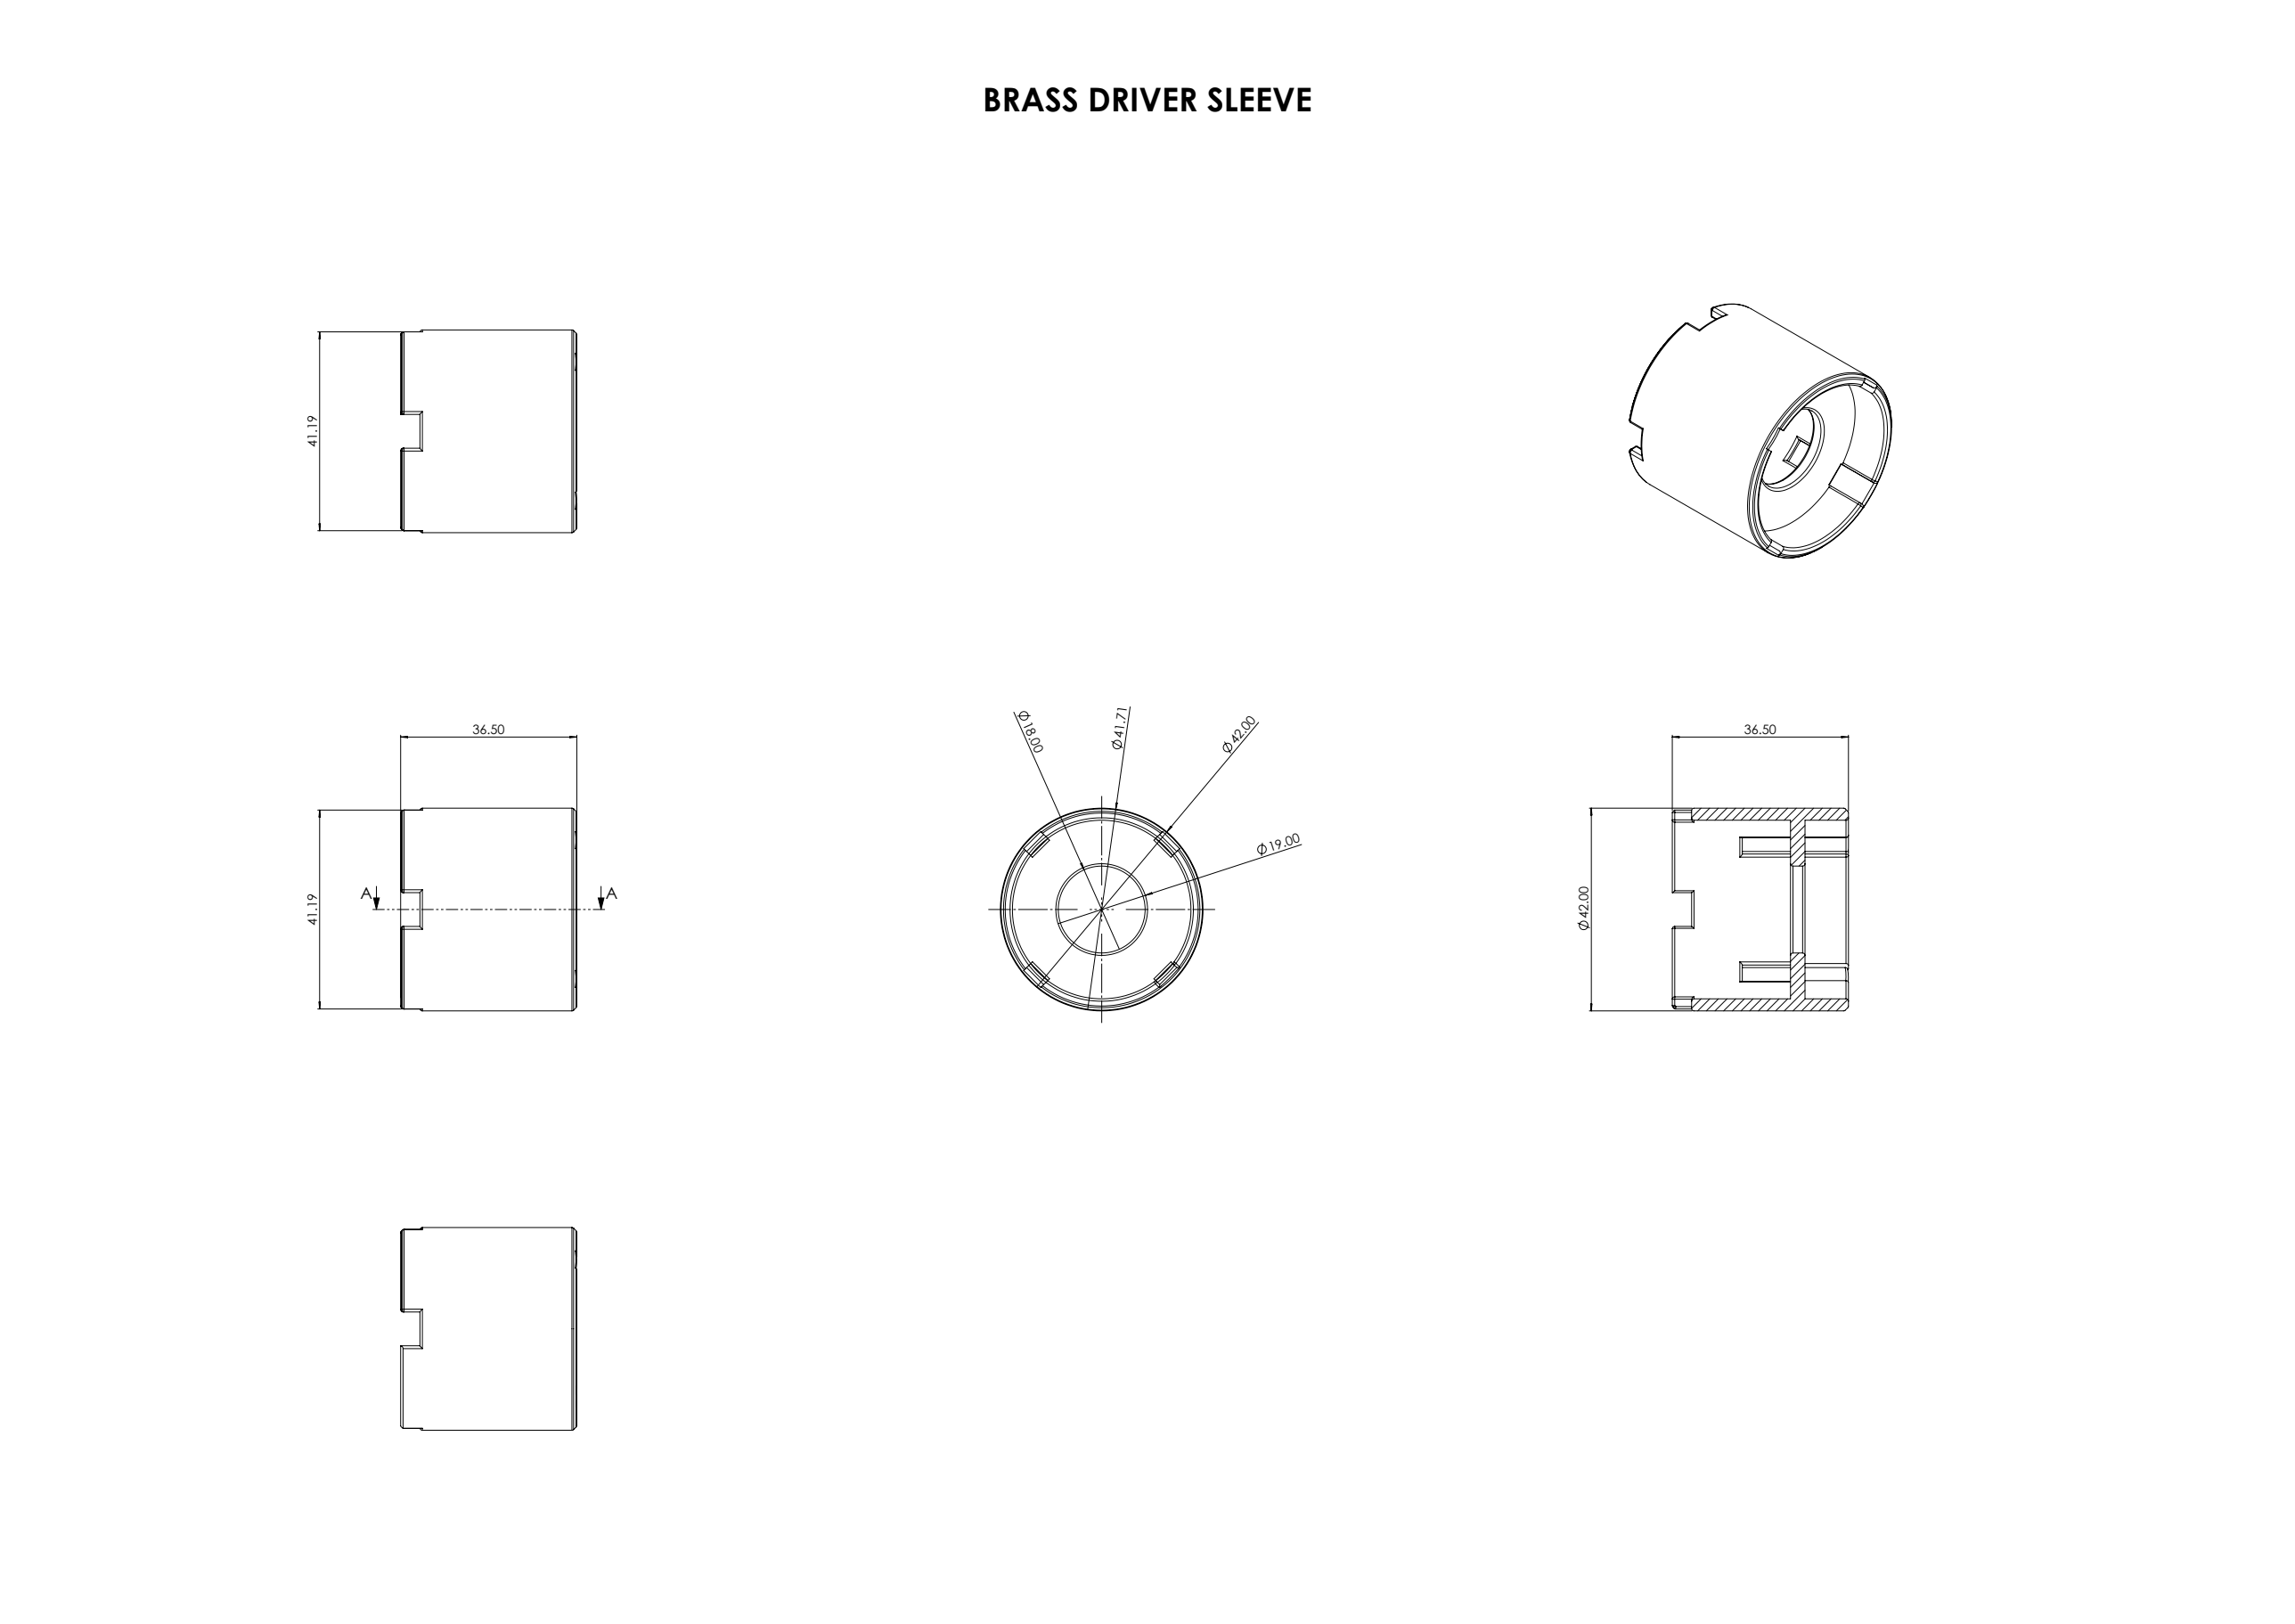
ISO-10303-21;
HEADER;
/* Generated by software containing ST-Developer
 * from STEP Tools, Inc. (www.steptools.com) 
 */

FILE_DESCRIPTION(
/* description */ (''),
/* implementation_level */ '2;1');

FILE_NAME(
/* name */ '11_Brass_Driver_Sleeve.step',
/* time_stamp */ '2026-10-11T13:00:10-07:00',
/* author */ (''),
/* organization */ (''),
/* preprocessor_version */ 'ST-DEVELOPER v20.2',
/* originating_system */ 'Autodesk Translation Framework v15.15.0.0',
/* authorisation */ '');

FILE_SCHEMA (('AUTOMOTIVE_DESIGN { 1 0 10303 214 3 1 1 }'));
ENDSEC;

DATA;
#10=MECHANICAL_DESIGN_GEOMETRIC_PRESENTATION_REPRESENTATION('',(#368),#65563);
#168=TOROIDAL_SURFACE('',#22042,9.5,0.5);
#169=TOROIDAL_SURFACE('',#22064,9.5,0.5);
#170=TOROIDAL_SURFACE('',#22095,20.2928932188135,0.5);
#171=TOROIDAL_SURFACE('',#22125,20.5,0.5);
#172=TOROIDAL_SURFACE('',#22149,20.5,0.5);
#173=TOROIDAL_SURFACE('',#22154,20.2928932188135,0.5);
#174=TOROIDAL_SURFACE('',#22157,20.5,0.5);
#175=TOROIDAL_SURFACE('',#22166,20.5,0.5);
#176=TOROIDAL_SURFACE('',#22186,20.5,0.5);
#177=TOROIDAL_SURFACE('',#22207,20.5,0.5);
#178=TOROIDAL_SURFACE('',#22220,20.5,0.5);
#179=TOROIDAL_SURFACE('',#22225,19.,0.5);
#180=TOROIDAL_SURFACE('',#22227,19.,0.5);
#181=TOROIDAL_SURFACE('',#22231,19.,0.5);
#182=TOROIDAL_SURFACE('',#22248,19.,0.5);
#183=TOROIDAL_SURFACE('',#22252,19.,0.5);
#184=TOROIDAL_SURFACE('',#22256,19.,0.5);
#185=TOROIDAL_SURFACE('',#22263,19.,0.5);
#186=TOROIDAL_SURFACE('',#22264,19.,0.5);
#187=TOROIDAL_SURFACE('',#22265,19.,0.5);
#188=TOROIDAL_SURFACE('',#22275,20.2928932188135,0.5);
#189=TOROIDAL_SURFACE('',#22289,19.,0.5);
#190=TOROIDAL_SURFACE('',#22299,19.,0.5);
#191=TOROIDAL_SURFACE('',#22302,20.5,0.5);
#192=TOROIDAL_SURFACE('',#22320,19.,0.5);
#193=TOROIDAL_SURFACE('',#22331,19.9928932188135,0.5);
#194=TOROIDAL_SURFACE('',#22335,19.,0.5);
#195=TOROIDAL_SURFACE('',#22338,19.9928932188135,0.5);
#196=TOROIDAL_SURFACE('',#22342,19.,0.5);
#197=TOROIDAL_SURFACE('',#22348,19.,0.5);
#198=TOROIDAL_SURFACE('',#22361,19.9928932188135,0.5);
#199=TOROIDAL_SURFACE('',#22372,19.,0.5);
#241=ELLIPSE('',#22319,0.707106781186544,0.5);
#242=ELLIPSE('',#22352,0.70710678118655,0.5);
#314=SPHERICAL_SURFACE('',#22100,0.5);
#315=SPHERICAL_SURFACE('',#22106,0.5);
#316=SPHERICAL_SURFACE('',#22109,0.5);
#317=SPHERICAL_SURFACE('',#22121,0.5);
#318=SPHERICAL_SURFACE('',#22142,0.5);
#319=SPHERICAL_SURFACE('',#22145,0.5);
#320=SPHERICAL_SURFACE('',#22162,0.5);
#321=SPHERICAL_SURFACE('',#22170,0.5);
#322=SPHERICAL_SURFACE('',#22173,0.5);
#323=SPHERICAL_SURFACE('',#22176,0.5);
#324=SPHERICAL_SURFACE('',#22191,0.5);
#325=SPHERICAL_SURFACE('',#22193,0.5);
#326=SPHERICAL_SURFACE('',#22200,0.5);
#327=SPHERICAL_SURFACE('',#22209,0.5);
#328=SPHERICAL_SURFACE('',#22217,0.5);
#329=SPHERICAL_SURFACE('',#22233,0.5);
#330=SPHERICAL_SURFACE('',#22259,0.5);
#331=SPHERICAL_SURFACE('',#22271,0.5);
#332=SPHERICAL_SURFACE('',#22282,0.500000000000002);
#333=SPHERICAL_SURFACE('',#22285,0.5);
#334=SPHERICAL_SURFACE('',#22324,0.5);
#335=SPHERICAL_SURFACE('',#22354,0.5);
#346=SHAPE_REPRESENTATION_RELATIONSHIP('SRR','None',#65624,#357);
#357=ADVANCED_BREP_SHAPE_REPRESENTATION('',(#379),#65562);
#368=STYLED_ITEM('',(#65802),#379);
#379=MANIFOLD_SOLID_BREP('Body1',#20018);
#495=CONICAL_SURFACE('',#22114,20.75,0.785398163397451);
#496=CONICAL_SURFACE('',#22152,20.75,0.785398163397451);
#497=CONICAL_SURFACE('',#22306,20.6,0.785398163397448);
#498=CONICAL_SURFACE('',#22380,20.75,0.785398163397451);
#499=CONICAL_SURFACE('',#22381,20.75,0.785398163397451);
#828=(
BOUNDED_CURVE()
B_SPLINE_CURVE(2,(#64727,#64728,#64729),.UNSPECIFIED.,.F.,.F.)
B_SPLINE_CURVE_WITH_KNOTS((3,3),(0.338124280435932,0.360943681531408),
 .UNSPECIFIED.)
CURVE()
GEOMETRIC_REPRESENTATION_ITEM()
RATIONAL_B_SPLINE_CURVE((1.00248873269084,1.00246071159709,1.00241757299052))
REPRESENTATION_ITEM('')
);
#829=(
BOUNDED_CURVE()
B_SPLINE_CURVE(2,(#64784,#64785,#64786),.UNSPECIFIED.,.F.,.F.)
B_SPLINE_CURVE_WITH_KNOTS((3,3),(0.230710993510061,0.25353039460556),
 .UNSPECIFIED.)
CURVE()
GEOMETRIC_REPRESENTATION_ITEM()
RATIONAL_B_SPLINE_CURVE((1.00241757299153,1.00246071159813,1.00248873269188))
REPRESENTATION_ITEM('')
);
#830=(
BOUNDED_CURVE()
B_SPLINE_CURVE(2,(#64793,#64794,#64795),.UNSPECIFIED.,.F.,.F.)
B_SPLINE_CURVE_WITH_KNOTS((3,3),(0.338124280435769,0.360943681531267),
 .UNSPECIFIED.)
CURVE()
GEOMETRIC_REPRESENTATION_ITEM()
RATIONAL_B_SPLINE_CURVE((1.00248873269167,1.00246071159791,1.00241757299132))
REPRESENTATION_ITEM('')
);
#831=(
BOUNDED_CURVE()
B_SPLINE_CURVE(2,(#64802,#64803,#64804),.UNSPECIFIED.,.F.,.F.)
B_SPLINE_CURVE_WITH_KNOTS((3,3),(0.230710993510149,0.253530394605615),
 .UNSPECIFIED.)
CURVE()
GEOMETRIC_REPRESENTATION_ITEM()
RATIONAL_B_SPLINE_CURVE((1.00241757299006,1.00246071159663,1.00248873269037))
REPRESENTATION_ITEM('')
);
#832=(
BOUNDED_CURVE()
B_SPLINE_CURVE(2,(#64812,#64813,#64814),.UNSPECIFIED.,.F.,.F.)
B_SPLINE_CURVE_WITH_KNOTS((3,3),(0.230710993510133,0.253530394605583),
 .UNSPECIFIED.)
CURVE()
GEOMETRIC_REPRESENTATION_ITEM()
RATIONAL_B_SPLINE_CURVE((1.00241757298939,1.00246071159594,1.00248873268967))
REPRESENTATION_ITEM('')
);
#833=(
BOUNDED_CURVE()
B_SPLINE_CURVE(2,(#64818,#64819,#64820),.UNSPECIFIED.,.F.,.F.)
B_SPLINE_CURVE_WITH_KNOTS((3,3),(0.338124280435993,0.360943681531517),
 .UNSPECIFIED.)
CURVE()
GEOMETRIC_REPRESENTATION_ITEM()
RATIONAL_B_SPLINE_CURVE((1.00248873269308,1.00246071159931,1.0024175729927))
REPRESENTATION_ITEM('')
);
#844=B_SPLINE_SURFACE_WITH_KNOTS('',3,3,((#63712,#63713,#63714,#63715),
(#63716,#63717,#63718,#63719),(#63720,#63721,#63722,#63723),(#63724,#63725,
#63726,#63727),(#63728,#63729,#63730,#63731),(#63732,#63733,#63734,#63735)),
 .UNSPECIFIED.,.F.,.F.,.F.,(4,1,1,4),(4,4),(0.,0.285714285714286,0.571428571428571,
1.),(0.143091562311917,0.172672323717935),.UNSPECIFIED.);
#845=B_SPLINE_SURFACE_WITH_KNOTS('',3,3,((#63754,#63755,#63756,#63757),
(#63758,#63759,#63760,#63761),(#63762,#63763,#63764,#63765),(#63766,#63767,
#63768,#63769),(#63770,#63771,#63772,#63773),(#63774,#63775,#63776,#63777)),
 .UNSPECIFIED.,.F.,.F.,.F.,(4,1,1,4),(4,4),(0.,0.285714285714286,0.571428571428571,
1.),(0.144052021996696,0.173632784471181),.UNSPECIFIED.);
#846=B_SPLINE_SURFACE_WITH_KNOTS('',3,3,((#63891,#63892,#63893,#63894),
(#63895,#63896,#63897,#63898),(#63899,#63900,#63901,#63902),(#63903,#63904,
#63905,#63906),(#63907,#63908,#63909,#63910),(#63911,#63912,#63913,#63914)),
 .UNSPECIFIED.,.F.,.F.,.F.,(4,1,1,4),(4,4),(0.,0.285714285714286,0.571428571428571,
1.),(0.357860307352845,0.38744106972591),.UNSPECIFIED.);
#847=B_SPLINE_SURFACE_WITH_KNOTS('',3,3,((#63991,#63992,#63993,#63994),
(#63995,#63996,#63997,#63998),(#63999,#64000,#64001,#64002),(#64003,#64004,
#64005,#64006),(#64007,#64008,#64009,#64010),(#64011,#64012,#64013,#64014)),
 .UNSPECIFIED.,.F.,.F.,.F.,(4,1,1,4),(4,4),(0.,0.285714285714286,0.571428571428571,
1.),(2.06363027950495E-16,0.0295807623344723),.UNSPECIFIED.);
#848=B_SPLINE_SURFACE_WITH_KNOTS('',3,3,((#64023,#64024,#64025,#64026),
(#64027,#64028,#64029,#64030),(#64031,#64032,#64033,#64034),(#64035,#64036,
#64037,#64038),(#64039,#64040,#64041,#64042),(#64043,#64044,#64045,#64046)),
 .UNSPECIFIED.,.F.,.F.,.F.,(4,1,1,4),(4,4),(0.,0.285714285714286,0.571428571428571,
1.),(6.08201692644882E-19,0.0295807623160019),.UNSPECIFIED.);
#849=B_SPLINE_SURFACE_WITH_KNOTS('',3,3,((#64167,#64168,#64169,#64170),
(#64171,#64172,#64173,#64174),(#64175,#64176,#64177,#64178),(#64179,#64180,
#64181,#64182),(#64183,#64184,#64185,#64186),(#64187,#64188,#64189,#64190)),
 .UNSPECIFIED.,.F.,.F.,.F.,(4,1,1,4),(4,4),(0.,0.285714285714286,0.571428571428571,
1.),(2.15031488595949E-16,0.0295807575131674),.UNSPECIFIED.);
#850=B_SPLINE_SURFACE_WITH_KNOTS('',3,3,((#65115,#65116,#65117,#65118),
(#65119,#65120,#65121,#65122),(#65123,#65124,#65125,#65126),(#65127,#65128,
#65129,#65130),(#65131,#65132,#65133,#65134),(#65135,#65136,#65137,#65138),
(#65139,#65140,#65141,#65142)),.UNSPECIFIED.,.F.,.F.,.F.,(4,1,1,1,4),(4,
4),(0.,0.285714285714286,0.571428571428571,0.857142857142857,1.),(0.82916884759973,
1.33025671401017),.UNSPECIFIED.);
#851=B_SPLINE_SURFACE_WITH_KNOTS('',3,3,((#65237,#65238,#65239,#65240),
(#65241,#65242,#65243,#65244),(#65245,#65246,#65247,#65248),(#65249,#65250,
#65251,#65252),(#65253,#65254,#65255,#65256),(#65257,#65258,#65259,#65260),
(#65261,#65262,#65263,#65264)),.UNSPECIFIED.,.F.,.F.,.F.,(4,1,1,1,4),(4,
4),(0.,0.285714285714286,0.571428571428571,0.857142857142857,1.),(0.829183372221167,
1.33027123863146),.UNSPECIFIED.);
#852=B_SPLINE_SURFACE_WITH_KNOTS('',3,3,((#65276,#65277,#65278,#65279),
(#65280,#65281,#65282,#65283),(#65284,#65285,#65286,#65287),(#65288,#65289,
#65290,#65291),(#65292,#65293,#65294,#65295),(#65296,#65297,#65298,#65299),
(#65300,#65301,#65302,#65303)),.UNSPECIFIED.,.F.,.F.,.F.,(4,1,1,1,4),(4,
4),(0.,0.285714285714286,0.571428571428571,0.857142857142857,1.),(0.829168847599735,
1.33025671401018),.UNSPECIFIED.);
#1040=PLANE('',#22050);
#1041=PLANE('',#22067);
#1042=PLANE('',#22077);
#1043=PLANE('',#22084);
#1044=PLANE('',#22091);
#1045=PLANE('',#22117);
#1046=PLANE('',#22123);
#1047=PLANE('',#22159);
#1048=PLANE('',#22183);
#1049=PLANE('',#22188);
#1050=PLANE('',#22197);
#1051=PLANE('',#22210);
#1052=PLANE('',#22213);
#1053=PLANE('',#22222);
#1054=PLANE('',#22250);
#1055=PLANE('',#22254);
#1056=PLANE('',#22267);
#1057=PLANE('',#22274);
#1058=PLANE('',#22278);
#1059=PLANE('',#22291);
#1060=PLANE('',#22292);
#1061=PLANE('',#22296);
#1062=PLANE('',#22298);
#1063=PLANE('',#22301);
#1064=PLANE('',#22312);
#1065=PLANE('',#22314);
#1066=PLANE('',#22316);
#1067=PLANE('',#22328);
#1068=PLANE('',#22330);
#1069=PLANE('',#22333);
#1070=PLANE('',#22337);
#1071=PLANE('',#22340);
#1072=PLANE('',#22344);
#1073=PLANE('',#22345);
#1074=PLANE('',#22358);
#1075=PLANE('',#22363);
#1076=PLANE('',#22366);
#1077=PLANE('',#22368);
#1078=PLANE('',#22374);
#1079=PLANE('',#22375);
#1080=PLANE('',#22376);
#1081=PLANE('',#22379);
#1124=FACE_BOUND('',#3382,.T.);
#1125=FACE_BOUND('',#3385,.T.);
#2151=FACE_OUTER_BOUND('',#3379,.T.);
#2152=FACE_OUTER_BOUND('',#3380,.T.);
#2153=FACE_OUTER_BOUND('',#3381,.T.);
#2154=FACE_OUTER_BOUND('',#3383,.T.);
#2155=FACE_OUTER_BOUND('',#3384,.T.);
#2156=FACE_OUTER_BOUND('',#3386,.T.);
#2157=FACE_OUTER_BOUND('',#3387,.T.);
#2158=FACE_OUTER_BOUND('',#3388,.T.);
#2159=FACE_OUTER_BOUND('',#3389,.T.);
#2160=FACE_OUTER_BOUND('',#3390,.T.);
#2161=FACE_OUTER_BOUND('',#3391,.T.);
#2162=FACE_OUTER_BOUND('',#3392,.T.);
#2163=FACE_OUTER_BOUND('',#3393,.T.);
#2164=FACE_OUTER_BOUND('',#3394,.T.);
#2165=FACE_OUTER_BOUND('',#3395,.T.);
#2166=FACE_OUTER_BOUND('',#3396,.T.);
#2167=FACE_OUTER_BOUND('',#3397,.T.);
#2168=FACE_OUTER_BOUND('',#3398,.T.);
#2169=FACE_OUTER_BOUND('',#3399,.T.);
#2170=FACE_OUTER_BOUND('',#3400,.T.);
#2171=FACE_OUTER_BOUND('',#3401,.T.);
#2172=FACE_OUTER_BOUND('',#3402,.T.);
#2173=FACE_OUTER_BOUND('',#3403,.T.);
#2174=FACE_OUTER_BOUND('',#3404,.T.);
#2175=FACE_OUTER_BOUND('',#3405,.T.);
#2176=FACE_OUTER_BOUND('',#3406,.T.);
#2177=FACE_OUTER_BOUND('',#3407,.T.);
#2178=FACE_OUTER_BOUND('',#3408,.T.);
#2179=FACE_OUTER_BOUND('',#3409,.T.);
#2180=FACE_OUTER_BOUND('',#3410,.T.);
#2181=FACE_OUTER_BOUND('',#3411,.T.);
#2182=FACE_OUTER_BOUND('',#3412,.T.);
#2183=FACE_OUTER_BOUND('',#3413,.T.);
#2184=FACE_OUTER_BOUND('',#3414,.T.);
#2185=FACE_OUTER_BOUND('',#3415,.T.);
#2186=FACE_OUTER_BOUND('',#3416,.T.);
#2187=FACE_OUTER_BOUND('',#3417,.T.);
#2188=FACE_OUTER_BOUND('',#3418,.T.);
#2189=FACE_OUTER_BOUND('',#3419,.T.);
#2190=FACE_OUTER_BOUND('',#3420,.T.);
#2191=FACE_OUTER_BOUND('',#3421,.T.);
#2192=FACE_OUTER_BOUND('',#3422,.T.);
#2193=FACE_OUTER_BOUND('',#3423,.T.);
#2194=FACE_OUTER_BOUND('',#3424,.T.);
#2195=FACE_OUTER_BOUND('',#3425,.T.);
#2196=FACE_OUTER_BOUND('',#3426,.T.);
#2197=FACE_OUTER_BOUND('',#3427,.T.);
#2198=FACE_OUTER_BOUND('',#3428,.T.);
#2199=FACE_OUTER_BOUND('',#3429,.T.);
#2200=FACE_OUTER_BOUND('',#3430,.T.);
#2201=FACE_OUTER_BOUND('',#3431,.T.);
#2202=FACE_OUTER_BOUND('',#3432,.T.);
#2203=FACE_OUTER_BOUND('',#3433,.T.);
#2204=FACE_OUTER_BOUND('',#3434,.T.);
#2205=FACE_OUTER_BOUND('',#3435,.T.);
#2206=FACE_OUTER_BOUND('',#3436,.T.);
#2207=FACE_OUTER_BOUND('',#3437,.T.);
#2208=FACE_OUTER_BOUND('',#3438,.T.);
#2209=FACE_OUTER_BOUND('',#3439,.T.);
#2210=FACE_OUTER_BOUND('',#3440,.T.);
#2211=FACE_OUTER_BOUND('',#3441,.T.);
#2212=FACE_OUTER_BOUND('',#3442,.T.);
#2213=FACE_OUTER_BOUND('',#3443,.T.);
#2214=FACE_OUTER_BOUND('',#3444,.T.);
#2215=FACE_OUTER_BOUND('',#3445,.T.);
#2216=FACE_OUTER_BOUND('',#3446,.T.);
#2217=FACE_OUTER_BOUND('',#3447,.T.);
#2218=FACE_OUTER_BOUND('',#3448,.T.);
#2219=FACE_OUTER_BOUND('',#3449,.T.);
#2220=FACE_OUTER_BOUND('',#3450,.T.);
#2221=FACE_OUTER_BOUND('',#3451,.T.);
#2222=FACE_OUTER_BOUND('',#3452,.T.);
#2223=FACE_OUTER_BOUND('',#3453,.T.);
#2224=FACE_OUTER_BOUND('',#3454,.T.);
#2225=FACE_OUTER_BOUND('',#3455,.T.);
#2226=FACE_OUTER_BOUND('',#3456,.T.);
#2227=FACE_OUTER_BOUND('',#3457,.T.);
#2228=FACE_OUTER_BOUND('',#3458,.T.);
#2229=FACE_OUTER_BOUND('',#3459,.T.);
#2230=FACE_OUTER_BOUND('',#3460,.T.);
#2231=FACE_OUTER_BOUND('',#3461,.T.);
#2232=FACE_OUTER_BOUND('',#3462,.T.);
#2233=FACE_OUTER_BOUND('',#3463,.T.);
#2234=FACE_OUTER_BOUND('',#3464,.T.);
#2235=FACE_OUTER_BOUND('',#3465,.T.);
#2236=FACE_OUTER_BOUND('',#3466,.T.);
#2237=FACE_OUTER_BOUND('',#3467,.T.);
#2238=FACE_OUTER_BOUND('',#3468,.T.);
#2239=FACE_OUTER_BOUND('',#3469,.T.);
#2240=FACE_OUTER_BOUND('',#3470,.T.);
#2241=FACE_OUTER_BOUND('',#3471,.T.);
#2242=FACE_OUTER_BOUND('',#3472,.T.);
#2243=FACE_OUTER_BOUND('',#3473,.T.);
#2244=FACE_OUTER_BOUND('',#3474,.T.);
#2245=FACE_OUTER_BOUND('',#3475,.T.);
#2246=FACE_OUTER_BOUND('',#3476,.T.);
#2247=FACE_OUTER_BOUND('',#3477,.T.);
#2248=FACE_OUTER_BOUND('',#3478,.T.);
#2249=FACE_OUTER_BOUND('',#3479,.T.);
#2250=FACE_OUTER_BOUND('',#3480,.T.);
#2251=FACE_OUTER_BOUND('',#3481,.T.);
#2252=FACE_OUTER_BOUND('',#3482,.T.);
#2253=FACE_OUTER_BOUND('',#3483,.T.);
#2254=FACE_OUTER_BOUND('',#3484,.T.);
#2255=FACE_OUTER_BOUND('',#3485,.T.);
#2256=FACE_OUTER_BOUND('',#3486,.T.);
#2257=FACE_OUTER_BOUND('',#3487,.T.);
#2258=FACE_OUTER_BOUND('',#3488,.T.);
#2259=FACE_OUTER_BOUND('',#3489,.T.);
#2260=FACE_OUTER_BOUND('',#3490,.T.);
#2261=FACE_OUTER_BOUND('',#3491,.T.);
#2262=FACE_OUTER_BOUND('',#3492,.T.);
#2263=FACE_OUTER_BOUND('',#3493,.T.);
#2264=FACE_OUTER_BOUND('',#3494,.T.);
#2265=FACE_OUTER_BOUND('',#3495,.T.);
#2266=FACE_OUTER_BOUND('',#3496,.T.);
#2267=FACE_OUTER_BOUND('',#3497,.T.);
#2268=FACE_OUTER_BOUND('',#3498,.T.);
#2269=FACE_OUTER_BOUND('',#3499,.T.);
#2270=FACE_OUTER_BOUND('',#3500,.T.);
#2271=FACE_OUTER_BOUND('',#3501,.T.);
#2272=FACE_OUTER_BOUND('',#3502,.T.);
#2273=FACE_OUTER_BOUND('',#3503,.T.);
#2274=FACE_OUTER_BOUND('',#3504,.T.);
#2275=FACE_OUTER_BOUND('',#3505,.T.);
#2276=FACE_OUTER_BOUND('',#3506,.T.);
#2277=FACE_OUTER_BOUND('',#3507,.T.);
#2278=FACE_OUTER_BOUND('',#3508,.T.);
#2279=FACE_OUTER_BOUND('',#3509,.T.);
#2280=FACE_OUTER_BOUND('',#3510,.T.);
#2281=FACE_OUTER_BOUND('',#3511,.T.);
#2282=FACE_OUTER_BOUND('',#3512,.T.);
#2283=FACE_OUTER_BOUND('',#3513,.T.);
#2284=FACE_OUTER_BOUND('',#3514,.T.);
#2285=FACE_OUTER_BOUND('',#3515,.T.);
#2286=FACE_OUTER_BOUND('',#3516,.T.);
#2287=FACE_OUTER_BOUND('',#3517,.T.);
#2288=FACE_OUTER_BOUND('',#3518,.T.);
#2289=FACE_OUTER_BOUND('',#3519,.T.);
#2290=FACE_OUTER_BOUND('',#3520,.T.);
#2291=FACE_OUTER_BOUND('',#3521,.T.);
#2292=FACE_OUTER_BOUND('',#3522,.T.);
#2293=FACE_OUTER_BOUND('',#3523,.T.);
#2294=FACE_OUTER_BOUND('',#3524,.T.);
#2295=FACE_OUTER_BOUND('',#3525,.T.);
#2296=FACE_OUTER_BOUND('',#3526,.T.);
#2297=FACE_OUTER_BOUND('',#3527,.T.);
#2298=FACE_OUTER_BOUND('',#3528,.T.);
#2299=FACE_OUTER_BOUND('',#3529,.T.);
#2300=FACE_OUTER_BOUND('',#3530,.T.);
#2301=FACE_OUTER_BOUND('',#3531,.T.);
#2302=FACE_OUTER_BOUND('',#3532,.T.);
#2303=FACE_OUTER_BOUND('',#3533,.T.);
#2304=FACE_OUTER_BOUND('',#3534,.T.);
#2305=FACE_OUTER_BOUND('',#3535,.T.);
#2306=FACE_OUTER_BOUND('',#3536,.T.);
#2307=FACE_OUTER_BOUND('',#3537,.T.);
#2308=FACE_OUTER_BOUND('',#3538,.T.);
#2309=FACE_OUTER_BOUND('',#3539,.T.);
#2310=FACE_OUTER_BOUND('',#3540,.T.);
#2311=FACE_OUTER_BOUND('',#3541,.T.);
#3379=EDGE_LOOP('',(#17440,#17441,#17442,#17443,#17444));
#3380=EDGE_LOOP('',(#17445,#17446,#17447,#17448,#17449,#17450));
#3381=EDGE_LOOP('',(#17451,#17452,#17453,#17454,#17455,#17456,#17457,#17458,
#17459,#17460,#17461,#17462,#17463,#17464,#17465,#17466,#17467,#17468,#17469,
#17470,#17471,#17472,#17473,#17474,#17475));
#3382=EDGE_LOOP('',(#17476));
#3383=EDGE_LOOP('',(#17477,#17478,#17479,#17480,#17481));
#3384=EDGE_LOOP('',(#17482,#17483,#17484,#17485,#17486,#17487,#17488,#17489,
#17490,#17491,#17492,#17493,#17494,#17495,#17496,#17497,#17498,#17499));
#3385=EDGE_LOOP('',(#17500));
#3386=EDGE_LOOP('',(#17501,#17502,#17503,#17504));
#3387=EDGE_LOOP('',(#17505,#17506,#17507,#17508));
#3388=EDGE_LOOP('',(#17509,#17510,#17511,#17512));
#3389=EDGE_LOOP('',(#17513,#17514,#17515,#17516));
#3390=EDGE_LOOP('',(#17517,#17518,#17519,#17520));
#3391=EDGE_LOOP('',(#17521,#17522,#17523,#17524));
#3392=EDGE_LOOP('',(#17525,#17526,#17527,#17528));
#3393=EDGE_LOOP('',(#17529,#17530,#17531,#17532));
#3394=EDGE_LOOP('',(#17533,#17534,#17535,#17536));
#3395=EDGE_LOOP('',(#17537,#17538,#17539,#17540));
#3396=EDGE_LOOP('',(#17541,#17542,#17543));
#3397=EDGE_LOOP('',(#17544,#17545,#17546,#17547));
#3398=EDGE_LOOP('',(#17548,#17549,#17550));
#3399=EDGE_LOOP('',(#17551,#17552,#17553));
#3400=EDGE_LOOP('',(#17554,#17555,#17556,#17557));
#3401=EDGE_LOOP('',(#17558,#17559,#17560,#17561));
#3402=EDGE_LOOP('',(#17562,#17563,#17564,#17565));
#3403=EDGE_LOOP('',(#17566,#17567,#17568,#17569));
#3404=EDGE_LOOP('',(#17570,#17571,#17572,#17573,#17574,#17575));
#3405=EDGE_LOOP('',(#17576,#17577,#17578,#17579,#17580));
#3406=EDGE_LOOP('',(#17581,#17582,#17583));
#3407=EDGE_LOOP('',(#17584,#17585,#17586,#17587));
#3408=EDGE_LOOP('',(#17588,#17589,#17590,#17591));
#3409=EDGE_LOOP('',(#17592,#17593,#17594,#17595,#17596,#17597,#17598,#17599,
#17600,#17601,#17602,#17603,#17604,#17605,#17606,#17607,#17608,#17609,#17610,
#17611,#17612));
#3410=EDGE_LOOP('',(#17613,#17614,#17615,#17616,#17617));
#3411=EDGE_LOOP('',(#17618,#17619,#17620));
#3412=EDGE_LOOP('',(#17621,#17622,#17623));
#3413=EDGE_LOOP('',(#17624,#17625,#17626,#17627));
#3414=EDGE_LOOP('',(#17628,#17629,#17630,#17631));
#3415=EDGE_LOOP('',(#17632,#17633,#17634,#17635));
#3416=EDGE_LOOP('',(#17636,#17637,#17638,#17639));
#3417=EDGE_LOOP('',(#17640,#17641,#17642,#17643));
#3418=EDGE_LOOP('',(#17644,#17645,#17646,#17647,#17648,#17649));
#3419=EDGE_LOOP('',(#17650,#17651,#17652));
#3420=EDGE_LOOP('',(#17653,#17654,#17655,#17656));
#3421=EDGE_LOOP('',(#17657,#17658,#17659));
#3422=EDGE_LOOP('',(#17660,#17661,#17662));
#3423=EDGE_LOOP('',(#17663,#17664,#17665));
#3424=EDGE_LOOP('',(#17666,#17667,#17668,#17669));
#3425=EDGE_LOOP('',(#17670,#17671,#17672,#17673));
#3426=EDGE_LOOP('',(#17674,#17675,#17676,#17677,#17678));
#3427=EDGE_LOOP('',(#17679,#17680,#17681,#17682,#17683));
#3428=EDGE_LOOP('',(#17684,#17685,#17686,#17687,#17688,#17689));
#3429=EDGE_LOOP('',(#17690,#17691,#17692,#17693));
#3430=EDGE_LOOP('',(#17694,#17695,#17696,#17697,#17698));
#3431=EDGE_LOOP('',(#17699,#17700,#17701,#17702,#17703,#17704));
#3432=EDGE_LOOP('',(#17705,#17706,#17707));
#3433=EDGE_LOOP('',(#17708,#17709,#17710));
#3434=EDGE_LOOP('',(#17711,#17712,#17713,#17714));
#3435=EDGE_LOOP('',(#17715,#17716,#17717,#17718,#17719,#17720));
#3436=EDGE_LOOP('',(#17721,#17722,#17723,#17724,#17725));
#3437=EDGE_LOOP('',(#17726,#17727,#17728));
#3438=EDGE_LOOP('',(#17729,#17730,#17731,#17732));
#3439=EDGE_LOOP('',(#17733,#17734,#17735,#17736,#17737));
#3440=EDGE_LOOP('',(#17738,#17739,#17740,#17741));
#3441=EDGE_LOOP('',(#17742,#17743,#17744));
#3442=EDGE_LOOP('',(#17745,#17746,#17747,#17748,#17749,#17750));
#3443=EDGE_LOOP('',(#17751,#17752,#17753,#17754));
#3444=EDGE_LOOP('',(#17755,#17756,#17757,#17758));
#3445=EDGE_LOOP('',(#17759,#17760,#17761,#17762));
#3446=EDGE_LOOP('',(#17763,#17764,#17765));
#3447=EDGE_LOOP('',(#17766,#17767,#17768,#17769));
#3448=EDGE_LOOP('',(#17770,#17771,#17772,#17773,#17774,#17775));
#3449=EDGE_LOOP('',(#17776,#17777,#17778,#17779,#17780,#17781));
#3450=EDGE_LOOP('',(#17782,#17783,#17784,#17785));
#3451=EDGE_LOOP('',(#17786,#17787,#17788,#17789));
#3452=EDGE_LOOP('',(#17790,#17791,#17792,#17793,#17794,#17795));
#3453=EDGE_LOOP('',(#17796,#17797,#17798));
#3454=EDGE_LOOP('',(#17799,#17800,#17801,#17802));
#3455=EDGE_LOOP('',(#17803,#17804,#17805,#17806,#17807,#17808,#17809,#17810,
#17811,#17812,#17813,#17814,#17815,#17816,#17817,#17818,#17819,#17820,#17821,
#17822,#17823,#17824,#17825,#17826,#17827,#17828,#17829,#17830,#17831,#17832,
#17833,#17834,#17835,#17836,#17837,#17838));
#3456=EDGE_LOOP('',(#17839,#17840,#17841,#17842));
#3457=EDGE_LOOP('',(#17843,#17844,#17845,#17846,#17847,#17848));
#3458=EDGE_LOOP('',(#17849,#17850,#17851,#17852));
#3459=EDGE_LOOP('',(#17853,#17854,#17855,#17856));
#3460=EDGE_LOOP('',(#17857,#17858,#17859,#17860,#17861,#17862));
#3461=EDGE_LOOP('',(#17863,#17864,#17865,#17866));
#3462=EDGE_LOOP('',(#17867,#17868,#17869,#17870));
#3463=EDGE_LOOP('',(#17871,#17872,#17873,#17874,#17875));
#3464=EDGE_LOOP('',(#17876,#17877,#17878));
#3465=EDGE_LOOP('',(#17879,#17880,#17881,#17882));
#3466=EDGE_LOOP('',(#17883,#17884,#17885,#17886,#17887,#17888,#17889));
#3467=EDGE_LOOP('',(#17890,#17891,#17892,#17893));
#3468=EDGE_LOOP('',(#17894,#17895,#17896,#17897,#17898,#17899));
#3469=EDGE_LOOP('',(#17900,#17901,#17902,#17903,#17904,#17905));
#3470=EDGE_LOOP('',(#17906,#17907,#17908,#17909));
#3471=EDGE_LOOP('',(#17910,#17911,#17912,#17913));
#3472=EDGE_LOOP('',(#17914,#17915,#17916));
#3473=EDGE_LOOP('',(#17917,#17918,#17919,#17920,#17921));
#3474=EDGE_LOOP('',(#17922,#17923,#17924,#17925,#17926));
#3475=EDGE_LOOP('',(#17927,#17928,#17929,#17930));
#3476=EDGE_LOOP('',(#17931,#17932,#17933,#17934));
#3477=EDGE_LOOP('',(#17935,#17936,#17937,#17938));
#3478=EDGE_LOOP('',(#17939,#17940,#17941));
#3479=EDGE_LOOP('',(#17942,#17943,#17944));
#3480=EDGE_LOOP('',(#17945,#17946,#17947,#17948));
#3481=EDGE_LOOP('',(#17949,#17950,#17951,#17952));
#3482=EDGE_LOOP('',(#17953,#17954,#17955,#17956));
#3483=EDGE_LOOP('',(#17957,#17958,#17959,#17960,#17961,#17962));
#3484=EDGE_LOOP('',(#17963,#17964,#17965,#17966,#17967));
#3485=EDGE_LOOP('',(#17968,#17969,#17970,#17971,#17972,#17973));
#3486=EDGE_LOOP('',(#17974,#17975,#17976,#17977,#17978,#17979));
#3487=EDGE_LOOP('',(#17980,#17981,#17982,#17983));
#3488=EDGE_LOOP('',(#17984,#17985,#17986,#17987,#17988,#17989,#17990,#17991,
#17992,#17993,#17994,#17995,#17996,#17997,#17998));
#3489=EDGE_LOOP('',(#17999,#18000,#18001,#18002,#18003,#18004));
#3490=EDGE_LOOP('',(#18005,#18006,#18007,#18008));
#3491=EDGE_LOOP('',(#18009,#18010,#18011,#18012,#18013,#18014));
#3492=EDGE_LOOP('',(#18015,#18016,#18017,#18018,#18019,#18020,#18021,#18022,
#18023,#18024,#18025,#18026,#18027,#18028,#18029,#18030,#18031));
#3493=EDGE_LOOP('',(#18032,#18033,#18034,#18035));
#3494=EDGE_LOOP('',(#18036,#18037,#18038,#18039,#18040,#18041,#18042,#18043,
#18044,#18045,#18046,#18047,#18048,#18049,#18050));
#3495=EDGE_LOOP('',(#18051,#18052,#18053,#18054));
#3496=EDGE_LOOP('',(#18055,#18056,#18057,#18058,#18059,#18060,#18061,#18062,
#18063,#18064,#18065,#18066,#18067,#18068,#18069));
#3497=EDGE_LOOP('',(#18070,#18071,#18072,#18073));
#3498=EDGE_LOOP('',(#18074,#18075,#18076,#18077,#18078,#18079,#18080,#18081,
#18082,#18083,#18084,#18085,#18086,#18087,#18088));
#3499=EDGE_LOOP('',(#18089,#18090,#18091,#18092,#18093));
#3500=EDGE_LOOP('',(#18094,#18095,#18096,#18097));
#3501=EDGE_LOOP('',(#18098,#18099,#18100));
#3502=EDGE_LOOP('',(#18101,#18102,#18103,#18104));
#3503=EDGE_LOOP('',(#18105,#18106,#18107,#18108));
#3504=EDGE_LOOP('',(#18109,#18110,#18111,#18112));
#3505=EDGE_LOOP('',(#18113,#18114,#18115,#18116));
#3506=EDGE_LOOP('',(#18117,#18118,#18119,#18120));
#3507=EDGE_LOOP('',(#18121,#18122,#18123,#18124));
#3508=EDGE_LOOP('',(#18125,#18126,#18127,#18128));
#3509=EDGE_LOOP('',(#18129,#18130,#18131,#18132));
#3510=EDGE_LOOP('',(#18133,#18134,#18135,#18136));
#3511=EDGE_LOOP('',(#18137,#18138,#18139,#18140));
#3512=EDGE_LOOP('',(#18141,#18142,#18143,#18144));
#3513=EDGE_LOOP('',(#18145,#18146,#18147,#18148));
#3514=EDGE_LOOP('',(#18149,#18150,#18151,#18152));
#3515=EDGE_LOOP('',(#18153,#18154,#18155,#18156));
#3516=EDGE_LOOP('',(#18157,#18158,#18159,#18160));
#3517=EDGE_LOOP('',(#18161,#18162,#18163,#18164));
#3518=EDGE_LOOP('',(#18165,#18166,#18167,#18168));
#3519=EDGE_LOOP('',(#18169,#18170,#18171,#18172,#18173));
#3520=EDGE_LOOP('',(#18174,#18175,#18176));
#3521=EDGE_LOOP('',(#18177,#18178,#18179,#18180));
#3522=EDGE_LOOP('',(#18181,#18182,#18183,#18184));
#3523=EDGE_LOOP('',(#18185,#18186,#18187,#18188,#18189,#18190,#18191,#18192,
#18193,#18194,#18195));
#3524=EDGE_LOOP('',(#18196,#18197,#18198,#18199,#18200,#18201,#18202,#18203,
#18204,#18205,#18206));
#3525=EDGE_LOOP('',(#18207,#18208,#18209,#18210,#18211,#18212));
#3526=EDGE_LOOP('',(#18213,#18214,#18215,#18216,#18217,#18218,#18219,#18220,
#18221,#18222,#18223));
#3527=EDGE_LOOP('',(#18224,#18225,#18226,#18227));
#3528=EDGE_LOOP('',(#18228,#18229,#18230,#18231));
#3529=EDGE_LOOP('',(#18232,#18233,#18234,#18235));
#3530=EDGE_LOOP('',(#18236,#18237,#18238,#18239));
#3531=EDGE_LOOP('',(#18240,#18241,#18242,#18243));
#3532=EDGE_LOOP('',(#18244,#18245,#18246,#18247));
#3533=EDGE_LOOP('',(#18248,#18249,#18250,#18251,#18252,#18253));
#3534=EDGE_LOOP('',(#18254,#18255,#18256,#18257));
#3535=EDGE_LOOP('',(#18258,#18259,#18260,#18261,#18262,#18263,#18264,#18265,
#18266,#18267,#18268,#18269,#18270,#18271,#18272));
#3536=EDGE_LOOP('',(#18273,#18274,#18275,#18276,#18277,#18278,#18279,#18280,
#18281,#18282,#18283,#18284,#18285,#18286,#18287));
#3537=EDGE_LOOP('',(#18288,#18289,#18290,#18291));
#3538=EDGE_LOOP('',(#18292,#18293,#18294,#18295));
#3539=EDGE_LOOP('',(#18296,#18297,#18298,#18299,#18300,#18301));
#3540=EDGE_LOOP('',(#18302,#18303,#18304,#18305));
#3541=EDGE_LOOP('',(#18306,#18307,#18308,#18309));
#4483=CIRCLE('',#22043,9.5);
#4484=CIRCLE('',#22044,0.5);
#4485=CIRCLE('',#22045,9.);
#4486=CIRCLE('',#22046,9.);
#4487=CIRCLE('',#22048,9.);
#4488=CIRCLE('',#22049,9.);
#4489=CIRCLE('',#22051,0.5);
#4490=CIRCLE('',#22052,18.5);
#4491=CIRCLE('',#22053,0.5);
#4492=CIRCLE('',#22054,0.5);
#4493=CIRCLE('',#22055,18.5);
#4494=CIRCLE('',#22056,18.5);
#4495=CIRCLE('',#22057,0.5);
#4496=CIRCLE('',#22058,0.5);
#4497=CIRCLE('',#22059,18.5);
#4498=CIRCLE('',#22060,0.5);
#4499=CIRCLE('',#22061,0.5);
#4500=CIRCLE('',#22062,18.5);
#4501=CIRCLE('',#22063,0.5);
#4502=CIRCLE('',#22065,0.5);
#4503=CIRCLE('',#22066,9.5);
#4504=CIRCLE('',#22068,18.5);
#4505=CIRCLE('',#22069,18.5);
#4506=CIRCLE('',#22070,18.5);
#4507=CIRCLE('',#22071,0.5);
#4508=CIRCLE('',#22072,0.5);
#4509=CIRCLE('',#22073,18.5);
#4510=CIRCLE('',#22075,0.5);
#4511=CIRCLE('',#22076,0.5);
#4512=CIRCLE('',#22079,0.5);
#4513=CIRCLE('',#22080,0.5);
#4514=CIRCLE('',#22082,0.5);
#4515=CIRCLE('',#22083,0.5);
#4516=CIRCLE('',#22086,0.5);
#4517=CIRCLE('',#22087,0.5);
#4518=CIRCLE('',#22089,0.5);
#4519=CIRCLE('',#22090,0.5);
#4520=CIRCLE('',#22093,0.5);
#4521=CIRCLE('',#22094,0.5);
#4522=CIRCLE('',#22096,0.5);
#4523=CIRCLE('',#22097,20.6464466094067);
#4524=CIRCLE('',#22098,0.500000000405903);
#4525=CIRCLE('',#22099,20.2928932188135);
#4526=CIRCLE('',#22101,0.500000000000001);
#4527=CIRCLE('',#22102,0.5);
#4528=CIRCLE('',#22104,0.5);
#4529=CIRCLE('',#22105,0.5);
#4530=CIRCLE('',#22107,0.5);
#4531=CIRCLE('',#22108,0.5);
#4532=CIRCLE('',#22110,0.5);
#4533=CIRCLE('',#22112,0.500000000000001);
#4534=CIRCLE('',#22113,0.500000000000002);
#4535=CIRCLE('',#22115,20.8535533905933);
#4536=CIRCLE('',#22116,0.5);
#4537=CIRCLE('',#22119,0.499999999999995);
#4538=CIRCLE('',#22120,0.5);
#4539=CIRCLE('',#22122,0.5);
#4540=CIRCLE('',#22124,19.);
#4541=CIRCLE('',#22126,21.);
#4542=CIRCLE('',#22127,0.500000000000004);
#4543=CIRCLE('',#22129,21.);
#4544=CIRCLE('',#22130,21.);
#4545=CIRCLE('',#22131,21.);
#4546=CIRCLE('',#22132,21.);
#4547=CIRCLE('',#22133,21.);
#4548=CIRCLE('',#22134,21.);
#4549=CIRCLE('',#22135,21.);
#4550=CIRCLE('',#22136,21.);
#4551=CIRCLE('',#22137,21.);
#4552=CIRCLE('',#22138,21.);
#4553=CIRCLE('',#22140,0.5);
#4554=CIRCLE('',#22141,0.5);
#4555=CIRCLE('',#22143,0.499999999999999);
#4556=CIRCLE('',#22144,0.5);
#4557=CIRCLE('',#22146,0.499999999999999);
#4558=CIRCLE('',#22147,0.5);
#4559=CIRCLE('',#22148,0.5);
#4560=CIRCLE('',#22150,20.8535533905933);
#4561=CIRCLE('',#22151,0.5);
#4562=CIRCLE('',#22153,20.6464466094067);
#4563=CIRCLE('',#22155,20.2928932188135);
#4564=CIRCLE('',#22156,0.5);
#4565=CIRCLE('',#22158,20.5);
#4566=CIRCLE('',#22160,0.5);
#4567=CIRCLE('',#22161,19.);
#4568=CIRCLE('',#22163,0.5);
#4569=CIRCLE('',#22164,0.5);
#4570=CIRCLE('',#22165,0.5);
#4571=CIRCLE('',#22167,0.499999999999996);
#4572=CIRCLE('',#22168,20.8535533905933);
#4573=CIRCLE('',#22169,0.499999999999996);
#4574=CIRCLE('',#22171,0.5);
#4575=CIRCLE('',#22172,0.5);
#4576=CIRCLE('',#22174,0.499999999999998);
#4577=CIRCLE('',#22175,0.5);
#4578=CIRCLE('',#22177,0.499999999999999);
#4579=CIRCLE('',#22178,0.5);
#4580=CIRCLE('',#22179,0.5);
#4581=CIRCLE('',#22181,0.5);
#4582=CIRCLE('',#22185,0.5);
#4583=CIRCLE('',#22187,20.5);
#4584=CIRCLE('',#22189,19.);
#4585=CIRCLE('',#22190,0.5);
#4586=CIRCLE('',#22192,0.5);
#4587=CIRCLE('',#22194,0.500000000000001);
#4588=CIRCLE('',#22195,0.5);
#4589=CIRCLE('',#22199,0.5);
#4590=CIRCLE('',#22201,0.5);
#4591=CIRCLE('',#22202,0.5);
#4592=CIRCLE('',#22203,0.5);
#4593=CIRCLE('',#22205,0.499999999999995);
#4594=CIRCLE('',#22206,0.5);
#4595=CIRCLE('',#22208,20.5);
#4596=CIRCLE('',#22212,0.5);
#4597=CIRCLE('',#22214,19.);
#4598=CIRCLE('',#22216,0.5);
#4599=CIRCLE('',#22218,0.5);
#4600=CIRCLE('',#22219,0.5);
#4601=CIRCLE('',#22221,20.5);
#4602=CIRCLE('',#22223,0.5);
#4603=CIRCLE('',#22224,19.);
#4604=CIRCLE('',#22226,18.5);
#4605=CIRCLE('',#22228,18.5);
#4606=CIRCLE('',#22229,0.500000000000003);
#4607=CIRCLE('',#22232,18.5);
#4608=CIRCLE('',#22234,0.5);
#4609=CIRCLE('',#22237,18.5);
#4610=CIRCLE('',#22238,18.5);
#4611=CIRCLE('',#22239,18.5);
#4612=CIRCLE('',#22240,18.5);
#4613=CIRCLE('',#22241,18.5);
#4614=CIRCLE('',#22242,18.5);
#4615=CIRCLE('',#22243,18.5);
#4616=CIRCLE('',#22244,18.5);
#4617=CIRCLE('',#22245,18.5);
#4618=CIRCLE('',#22246,18.5);
#4619=CIRCLE('',#22249,19.);
#4620=CIRCLE('',#22253,19.);
#4621=CIRCLE('',#22257,0.500000000000004);
#4622=CIRCLE('',#22258,19.);
#4623=CIRCLE('',#22260,0.500000000000001);
#4624=CIRCLE('',#22261,0.5);
#4625=CIRCLE('',#22266,19.);
#4626=CIRCLE('',#22270,0.500000000000001);
#4627=CIRCLE('',#22272,0.5);
#4628=CIRCLE('',#22276,20.2928932188135);
#4629=CIRCLE('',#22277,20.6464466094067);
#4630=CIRCLE('',#22279,19.);
#4631=CIRCLE('',#22281,0.5);
#4632=CIRCLE('',#22283,0.5);
#4633=CIRCLE('',#22284,0.500000000000002);
#4634=CIRCLE('',#22286,0.500000000000003);
#4635=CIRCLE('',#22287,0.5);
#4636=CIRCLE('',#22293,20.5);
#4637=CIRCLE('',#22294,0.5);
#4638=CIRCLE('',#22300,19.);
#4639=CIRCLE('',#22303,20.8535533905933);
#4640=CIRCLE('',#22304,20.8535533905933);
#4641=CIRCLE('',#22305,0.5);
#4642=CIRCLE('',#22307,20.3464466094067);
#4643=CIRCLE('',#22308,20.3464466094067);
#4644=CIRCLE('',#22309,20.3464466094067);
#4645=CIRCLE('',#22310,20.3464466094067);
#4646=CIRCLE('',#22318,0.499999999999998);
#4647=CIRCLE('',#22321,18.5);
#4648=CIRCLE('',#22322,0.500000000000001);
#4649=CIRCLE('',#22323,19.);
#4650=CIRCLE('',#22325,0.500000000000001);
#4651=CIRCLE('',#22329,19.9928932188135);
#4652=CIRCLE('',#22332,19.9928932188135);
#4653=CIRCLE('',#22334,19.);
#4654=CIRCLE('',#22336,18.5);
#4655=CIRCLE('',#22339,19.9928932188135);
#4656=CIRCLE('',#22341,19.);
#4657=CIRCLE('',#22343,18.5);
#4658=CIRCLE('',#22346,19.9928932188135);
#4659=CIRCLE('',#22347,19.);
#4660=CIRCLE('',#22349,0.499999999999998);
#4661=CIRCLE('',#22350,18.5);
#4662=CIRCLE('',#22353,0.499999999999999);
#4663=CIRCLE('',#22355,0.500000000000001);
#4664=CIRCLE('',#22359,0.5);
#4665=CIRCLE('',#22360,0.5);
#4666=CIRCLE('',#22364,0.5);
#4667=CIRCLE('',#22365,0.5);
#4668=CIRCLE('',#22373,19.);
#5357=B_SPLINE_CURVE_WITH_KNOTS('',3,(#63737,#63738,#63739,#63740),
 .UNSPECIFIED.,.F.,.F.,(4,4),(0.143091562311917,0.172672323717935),
 .UNSPECIFIED.);
#5358=B_SPLINE_CURVE_WITH_KNOTS('',3,(#63743,#63744,#63745,#63746),
 .UNSPECIFIED.,.F.,.F.,(4,4),(-0.172672323717935,-0.143091563390451),
 .UNSPECIFIED.);
#5359=B_SPLINE_CURVE_WITH_KNOTS('',3,(#63749,#63750,#63751,#63752),
 .UNSPECIFIED.,.F.,.F.,(4,4),(-0.173632784471181,-0.144052021996696),
 .UNSPECIFIED.);
#5360=B_SPLINE_CURVE_WITH_KNOTS('',3,(#63779,#63780,#63781,#63782),
 .UNSPECIFIED.,.F.,.F.,(4,4),(0.144052023091887,0.173632784471181),
 .UNSPECIFIED.);
#5361=B_SPLINE_CURVE_WITH_KNOTS('',3,(#63788,#63789,#63790,#63791),
 .UNSPECIFIED.,.F.,.F.,(4,4),(-0.224098351300682,-0.214549181227953),
 .UNSPECIFIED.);
#5362=B_SPLINE_CURVE_WITH_KNOTS('',3,(#63798,#63799,#63800,#63801,#63802,
#63803,#63804,#63805,#63806,#63807,#63808,#63809,#63810,#63811),
 .UNSPECIFIED.,.F.,.F.,(4,2,2,2,2,2,4),(-0.224745183165744,-0.224338209360955,
-0.195801564669302,-0.167421789000985,-0.142834461201585,-0.123828977041314,
-0.107197280907097),.UNSPECIFIED.);
#5363=B_SPLINE_CURVE_WITH_KNOTS('',3,(#63866,#63867,#63868,#63869,#63870,
#63871,#63872,#63873,#63874,#63875,#63876,#63877,#63878,#63879),
 .UNSPECIFIED.,.F.,.F.,(4,2,2,2,2,2,4),(-0.0960754972725223,-0.0824346759427748,
-0.066846944434569,-0.0466811511835726,-0.0234049052400428,0.,0.000333787781842202),
 .UNSPECIFIED.);
#5364=B_SPLINE_CURVE_WITH_KNOTS('',3,(#63915,#63916,#63917,#63918),
 .UNSPECIFIED.,.F.,.F.,(4,4),(0.357860307352845,0.38744106972591),
 .UNSPECIFIED.);
#5365=B_SPLINE_CURVE_WITH_KNOTS('',3,(#63919,#63920,#63921,#63922),
 .UNSPECIFIED.,.F.,.F.,(4,4),(-0.38744106972591,-0.357860307352845),
 .UNSPECIFIED.);
#5366=B_SPLINE_CURVE_WITH_KNOTS('',3,(#63930,#63931,#63932,#63933),
 .UNSPECIFIED.,.F.,.F.,(4,4),(-0.0295807575131674,-2.15031488595949E-16),
 .UNSPECIFIED.);
#5367=B_SPLINE_CURVE_WITH_KNOTS('',3,(#63940,#63941,#63942,#63943,#63944,
#63945,#63946,#63947,#63948,#63949,#63950,#63951,#63952,#63953),
 .UNSPECIFIED.,.F.,.F.,(4,2,2,2,2,2,4),(0.0949936904735385,0.109164132542672,
0.125358949984382,0.146855590277485,0.168423573252805,0.190934620475292,
0.191367837777155),.UNSPECIFIED.);
#5368=B_SPLINE_CURVE_WITH_KNOTS('',3,(#64015,#64016,#64017,#64018),
 .UNSPECIFIED.,.F.,.F.,(4,4),(-0.0295807623344723,-2.06363027950495E-16),
 .UNSPECIFIED.);
#5369=B_SPLINE_CURVE_WITH_KNOTS('',3,(#64019,#64020,#64021,#64022),
 .UNSPECIFIED.,.F.,.F.,(4,4),(2.06363027950495E-16,0.0295807623344723),
 .UNSPECIFIED.);
#5370=B_SPLINE_CURVE_WITH_KNOTS('',3,(#64047,#64048,#64049,#64050),
 .UNSPECIFIED.,.F.,.F.,(4,4),(-0.0295807623160019,-6.08201692644882E-19),
 .UNSPECIFIED.);
#5371=B_SPLINE_CURVE_WITH_KNOTS('',3,(#64051,#64052,#64053,#64054),
 .UNSPECIFIED.,.F.,.F.,(4,4),(6.08201692644882E-19,0.0295807623160019),
 .UNSPECIFIED.);
#5372=B_SPLINE_CURVE_WITH_KNOTS('',3,(#64057,#64058,#64059,#64060,#64061,
#64062,#64063,#64064,#64065,#64066,#64067,#64068,#64069,#64070),
 .UNSPECIFIED.,.F.,.F.,(4,2,2,2,2,2,4),(-0.00043336587833757,0.,0.0225187676075078,
0.044094147534689,0.0655981603120321,0.0817985319256877,0.0959738338873166),
 .UNSPECIFIED.);
#5373=B_SPLINE_CURVE_WITH_KNOTS('',3,(#64081,#64082,#64083,#64084),
 .UNSPECIFIED.,.F.,.F.,(4,4),(0.21454918194711,0.224098351300682),
 .UNSPECIFIED.);
#5374=B_SPLINE_CURVE_WITH_KNOTS('',3,(#64092,#64093,#64094,#64095,#64096,
#64097,#64098,#64099,#64100,#64101,#64102,#64103,#64104,#64105),
 .UNSPECIFIED.,.F.,.F.,(4,2,2,2,2,2,4),(-0.000433365878018287,0.,0.0225187676075679,
0.04409414753479,0.0655981603121373,0.081798531925792,0.0959738338874173),
 .UNSPECIFIED.);
#5375=B_SPLINE_CURVE_WITH_KNOTS('',3,(#64122,#64123,#64124,#64125,#64126,
#64127,#64128,#64129,#64130,#64131,#64132,#64133),.UNSPECIFIED.,.F.,.F.,
(4,2,2,2,2,4),(0.,0.0151014582898052,0.0345370073824244,0.058455076138778,
0.0839695268602519,0.0844093817034405),.UNSPECIFIED.);
#5376=B_SPLINE_CURVE_WITH_KNOTS('',3,(#64140,#64141,#64142,#64143),
 .UNSPECIFIED.,.F.,.F.,(4,4),(-0.084228764664281,-0.0746795945915525),
 .UNSPECIFIED.);
#5377=B_SPLINE_CURVE_WITH_KNOTS('',3,(#64146,#64147,#64148,#64149,#64150,
#64151,#64152,#64153,#64154,#64155,#64156,#64157,#64158,#64159,#64160,#64161),
 .UNSPECIFIED.,.F.,.F.,(4,2,2,2,2,2,2,4),(-0.000449799814571451,0.,0.0220871623056755,
0.0431506585070033,0.0650141873659196,0.0813775476367432,0.0955802995948401,
0.0959539671675678),.UNSPECIFIED.);
#5378=B_SPLINE_CURVE_WITH_KNOTS('',3,(#64193,#64194,#64195,#64196),
 .UNSPECIFIED.,.F.,.F.,(4,4),(2.15031488595949E-16,0.0295807575131674),
 .UNSPECIFIED.);
#5379=B_SPLINE_CURVE_WITH_KNOTS('',3,(#64203,#64204,#64205,#64206,#64207,
#64208,#64209,#64210,#64211,#64212,#64213,#64214,#64215,#64216),
 .UNSPECIFIED.,.F.,.F.,(4,2,2,2,2,2,4),(0.,0.014053468854056,0.0301647070840401,
0.0516306547628395,0.0728079263494303,0.0950476067985505,0.0954931369347626),
 .UNSPECIFIED.);
#5380=B_SPLINE_CURVE_WITH_KNOTS('',3,(#64226,#64227,#64228,#64229),
 .UNSPECIFIED.,.F.,.F.,(4,4),(-0.224098351300682,-0.214549181227954),
 .UNSPECIFIED.);
#5381=B_SPLINE_CURVE_WITH_KNOTS('',3,(#64249,#64250,#64251,#64252,#64253,
#64254,#64255,#64256,#64257,#64258,#64259,#64260,#64261,#64262),
 .UNSPECIFIED.,.F.,.F.,(4,2,2,2,2,2,4),(0.0949936904735942,0.109164132542739,
0.125358949984464,0.146855590277593,0.168423573252929,0.190934620475441,
0.191367837777403),.UNSPECIFIED.);
#5382=B_SPLINE_CURVE_WITH_KNOTS('',3,(#64275,#64276,#64277,#64278,#64279,
#64280,#64281,#64282,#64283,#64284,#64285,#64286),.UNSPECIFIED.,.F.,.F.,
(4,2,2,2,2,4),(-0.000399537795305727,0.,0.0380148222930731,0.0673927529984265,
0.0894121467178007,0.0947714478271359),.UNSPECIFIED.);
#5383=B_SPLINE_CURVE_WITH_KNOTS('',3,(#64290,#64291,#64292,#64293,#64294,
#64295,#64296,#64297,#64298,#64299,#64300,#64301),.UNSPECIFIED.,.F.,.F.,
(4,2,2,2,2,4),(0.106231153334496,0.110609380645274,0.128597903585479,0.152597909542381,
0.183653737492122,0.183980135888318),.UNSPECIFIED.);
#5384=B_SPLINE_CURVE_WITH_KNOTS('',3,(#64302,#64303,#64304,#64305),
 .UNSPECIFIED.,.F.,.F.,(4,4),(0.0746795945915525,0.0842287639451254),
 .UNSPECIFIED.);
#5385=B_SPLINE_CURVE_WITH_KNOTS('',3,(#64306,#64307,#64308,#64309),
 .UNSPECIFIED.,.F.,.F.,(4,4),(0.21454918194711,0.224098351300682),
 .UNSPECIFIED.);
#5386=B_SPLINE_CURVE_WITH_KNOTS('',3,(#64318,#64319,#64320,#64321,#64322,
#64323,#64324,#64325,#64326,#64327,#64328,#64329),.UNSPECIFIED.,.F.,.F.,
(4,2,2,2,2,4),(0.,0.0151014582898128,0.0345370073824547,0.0584550761388158,
0.0839695268603532,0.0844093817034856),.UNSPECIFIED.);
#5387=B_SPLINE_CURVE_WITH_KNOTS('',3,(#64333,#64334,#64335,#64336,#64337,
#64338,#64339,#64340,#64341,#64342,#64343,#64344),.UNSPECIFIED.,.F.,.F.,
(4,2,2,2,2,4),(-0.000399537795187636,0.,0.0380148222927662,0.0673927529975771,
0.0894121467165036,0.0947714478257393),.UNSPECIFIED.);
#5388=B_SPLINE_CURVE_WITH_KNOTS('',3,(#64346,#64347,#64348,#64349),
 .UNSPECIFIED.,.F.,.F.,(4,4),(-0.084228764664281,-0.0746795945915525),
 .UNSPECIFIED.);
#5389=B_SPLINE_CURVE_WITH_KNOTS('',3,(#64355,#64356,#64357,#64358,#64359,
#64360,#64361,#64362,#64363,#64364,#64365,#64366),.UNSPECIFIED.,.F.,.F.,
(4,2,2,2,2,4),(-0.000444101878230381,0.,0.0380815409708187,0.0676748364114729,
0.0897163855403829,0.0947742742230686),.UNSPECIFIED.);
#5390=B_SPLINE_CURVE_WITH_KNOTS('',3,(#64410,#64411,#64412,#64413,#64414,
#64415,#64416,#64417,#64418,#64419,#64420,#64421),.UNSPECIFIED.,.F.,.F.,
(4,2,2,2,2,4),(-0.000444101878323987,0.,0.0380815409760417,0.0676748364256351,
0.0897163855612856,0.0981715128747534),.UNSPECIFIED.);
#5391=B_SPLINE_CURVE_WITH_KNOTS('',3,(#64424,#64425,#64426,#64427,#64428,
#64429,#64430,#64431,#64432,#64433,#64434,#64435),.UNSPECIFIED.,.F.,.F.,
(4,2,2,2,2,4),(0.103458653410514,0.110599336947648,0.128587640292216,0.152592542525185,
0.183648506748048,0.18397598979878),.UNSPECIFIED.);
#5392=B_SPLINE_CURVE_WITH_KNOTS('',3,(#64437,#64438,#64439,#64440),
 .UNSPECIFIED.,.F.,.F.,(4,4),(0.0743659931772117,0.08135049123277),
 .UNSPECIFIED.);
#5393=B_SPLINE_CURVE_WITH_KNOTS('',3,(#64443,#64444,#64445,#64446),
 .UNSPECIFIED.,.F.,.F.,(4,4),(-0.223127503799962,-0.216143005636944),
 .UNSPECIFIED.);
#5394=B_SPLINE_CURVE_WITH_KNOTS('',3,(#64456,#64457,#64458,#64459,#64460,
#64461,#64462,#64463,#64464,#64465,#64466,#64467),.UNSPECIFIED.,.F.,.F.,
(4,2,2,2,2,4),(-0.000444101878259206,0.,0.0380815409762479,0.0676748364260828,
0.089716385561879,0.0981715128754566),.UNSPECIFIED.);
#5395=B_SPLINE_CURVE_WITH_KNOTS('',3,(#64470,#64471,#64472,#64473,#64474,
#64475,#64476,#64477,#64478,#64479,#64480,#64481),.UNSPECIFIED.,.F.,.F.,
(4,2,2,2,2,4),(0.103458653410644,0.110599336947805,0.128587640292406,0.15259254252545,
0.183648506748331,0.18397598979916),.UNSPECIFIED.);
#5396=B_SPLINE_CURVE_WITH_KNOTS('',3,(#64483,#64484,#64485,#64486),
 .UNSPECIFIED.,.F.,.F.,(4,4),(0.0743659931772121,0.0813504912327701),
 .UNSPECIFIED.);
#5397=B_SPLINE_CURVE_WITH_KNOTS('',3,(#64489,#64490,#64491,#64492),
 .UNSPECIFIED.,.F.,.F.,(4,4),(-0.223127503799961,-0.216143005636943),
 .UNSPECIFIED.);
#5398=B_SPLINE_CURVE_WITH_KNOTS('',3,(#64500,#64501,#64502,#64503,#64504,
#64505,#64506,#64507,#64508,#64509,#64510,#64511),.UNSPECIFIED.,.F.,.F.,
(4,2,2,2,2,4),(-0.00044410187825338,0.,0.0380815409761677,0.0676748364257858,
0.0897163855613554,0.0947742742458168),.UNSPECIFIED.);
#5399=B_SPLINE_CURVE_WITH_KNOTS('',3,(#64518,#64519,#64520,#64521),
 .UNSPECIFIED.,.F.,.F.,(4,4),(0.0746795945915525,0.0842287646642811),
 .UNSPECIFIED.);
#5400=B_SPLINE_CURVE_WITH_KNOTS('',3,(#64522,#64523,#64524,#64525,#64526,
#64527,#64528,#64529,#64530,#64531,#64532,#64533),.UNSPECIFIED.,.F.,.F.,
(4,2,2,2,2,4),(0.,0.0151014582898057,0.0345370073824282,0.0584550761387909,
0.0839695268602773,0.084409381703446),.UNSPECIFIED.);
#5401=B_SPLINE_CURVE_WITH_KNOTS('',3,(#64541,#64542,#64543,#64544,#64545,
#64546,#64547,#64548,#64549,#64550,#64551,#64552),.UNSPECIFIED.,.F.,.F.,
(4,2,2,2,2,4),(0.,0.0151014582898054,0.0345370073824249,0.0584550761387796,
0.0839695268602591,0.0844093817034706),.UNSPECIFIED.);
#5402=B_SPLINE_CURVE_WITH_KNOTS('',3,(#64554,#64555,#64556,#64557),
 .UNSPECIFIED.,.F.,.F.,(4,4),(-0.0842287646642811,-0.0746795945915525),
 .UNSPECIFIED.);
#5403=B_SPLINE_CURVE_WITH_KNOTS('',3,(#64571,#64572,#64573,#64574,#64575,
#64576,#64577,#64578,#64579,#64580,#64581,#64582,#64583,#64584,#64585,#64586,
#64587,#64588,#64589,#64590,#64591),.UNSPECIFIED.,.F.,.F.,(4,2,2,2,2,3,
2,2,2,4),(0.158319501107787,0.167251782267889,0.176184063427991,0.187124730842742,
0.199384896436401,0.211645062030061,0.22379953303083,0.2359540040316,0.246692006811033,
0.264142032122818),.UNSPECIFIED.);
#5404=B_SPLINE_CURVE_WITH_KNOTS('',3,(#64625,#64626,#64627,#64628,#64629,
#64630,#64631,#64632,#64633,#64634,#64635,#64636),.UNSPECIFIED.,.F.,.F.,
(4,2,2,2,2,4),(0.181384150825648,0.206078531962836,0.231632932915096,0.252637853635304,
0.263140313995408,0.273642774355512),.UNSPECIFIED.);
#5405=B_SPLINE_CURVE_WITH_KNOTS('',3,(#64641,#64642,#64643,#64644,#64645,
#64646,#64647,#64648,#64649,#64650,#64651,#64652),.UNSPECIFIED.,.F.,.F.,
(4,2,2,2,2,4),(-0.0876802602836453,-0.0733239775103818,-0.0560578353470276,
-0.0325387048074095,0.,0.000330498359414059),.UNSPECIFIED.);
#5406=B_SPLINE_CURVE_WITH_KNOTS('',3,(#64656,#64657,#64658,#64659),
 .UNSPECIFIED.,.F.,.F.,(4,4),(0.216143005618354,0.223127503799962),
 .UNSPECIFIED.);
#5407=B_SPLINE_CURVE_WITH_KNOTS('',3,(#64665,#64666,#64667,#64668,#64669,
#64670,#64671,#64672,#64673,#64674,#64675,#64676,#64677,#64678,#64679,#64680,
#64681,#64682,#64683,#64684,#64685,#64686,#64687,#64688,#64689,#64690,#64691,
#64692,#64693,#64694,#64695,#64696,#64697,#64698,#64699,#64700,#64701,#64702,
#64703,#64704,#64705,#64706,#64707,#64708,#64709,#64710,#64711,#64712,#64713,
#64714,#64715,#64716,#64717,#64718,#64719,#64720,#64721,#64722,#64723,#64724,
#64725),.UNSPECIFIED.,.F.,.F.,(4,3,3,3,3,3,3,3,3,3,3,3,3,3,3,3,3,3,3,3,
4),(0.,0.00788945390620161,0.0159107528337136,0.0198233466742012,0.0278090397100955,
0.0338830033914972,0.0395609471880743,0.0474955046467764,0.0554321605872608,
0.0591436409533912,0.0671079528129928,0.0676235550484229,0.075592682599463,
0.0785910514609892,0.0865300392579837,0.0944439925209208,0.0979951919099392,
0.101302747945548,0.108060095589035,0.116004888439858,0.118137330218053),
 .UNSPECIFIED.);
#5408=B_SPLINE_CURVE_WITH_KNOTS('',3,(#64731,#64732,#64733,#64734,#64735,
#64736),.UNSPECIFIED.,.F.,.F.,(4,2,4),(0.0370807285215095,0.0556314474159261,
0.0743351338524323),.UNSPECIFIED.);
#5409=B_SPLINE_CURVE_WITH_KNOTS('',3,(#64740,#64741,#64742,#64743,#64744,
#64745,#64746,#64747,#64748,#64749),.UNSPECIFIED.,.F.,.F.,(4,2,2,2,4),(0.148746748488587,
0.167205194290617,0.185750729133706,0.204398921478351,0.223127503799962),
 .UNSPECIFIED.);
#5410=B_SPLINE_CURVE_WITH_KNOTS('',3,(#64754,#64755,#64756,#64757),
 .UNSPECIFIED.,.F.,.F.,(4,4),(0.0743659931772123,0.0813504912327697),
 .UNSPECIFIED.);
#5411=B_SPLINE_CURVE_WITH_KNOTS('',3,(#64759,#64760,#64761,#64762,#64763,
#64764,#64765,#64766,#64767,#64768,#64769,#64770),.UNSPECIFIED.,.F.,.F.,
(4,2,2,2,2,4),(0.103458653410611,0.110599336946118,0.128587640290153,0.152592542522104,
0.183648506743288,0.183975989794056),.UNSPECIFIED.);
#5412=B_SPLINE_CURVE_WITH_KNOTS('',3,(#64797,#64798,#64799,#64800),
 .UNSPECIFIED.,.F.,.F.,(4,4),(-1.32591570645538,-0.833509855154531),
 .UNSPECIFIED.);
#5413=B_SPLINE_CURVE_WITH_KNOTS('',3,(#64807,#64808,#64809,#64810),
 .UNSPECIFIED.,.F.,.F.,(4,4),(-1.32593023123408,-0.833524379933391),
 .UNSPECIFIED.);
#5414=B_SPLINE_CURVE_WITH_KNOTS('',3,(#64821,#64822,#64823,#64824),
 .UNSPECIFIED.,.F.,.F.,(4,4),(-1.32591570645538,-0.833509855154526),
 .UNSPECIFIED.);
#5415=B_SPLINE_CURVE_WITH_KNOTS('',3,(#64831,#64832,#64833,#64834,#64835,
#64836,#64837,#64838,#64839,#64840),.UNSPECIFIED.,.F.,.F.,(4,2,2,2,4),(0.0743659931772121,
0.0930945754988228,0.111742767843467,0.130288302686557,0.148746748488587),
 .UNSPECIFIED.);
#5416=B_SPLINE_CURVE_WITH_KNOTS('',3,(#64843,#64844,#64845,#64846,#64847,
#64848),.UNSPECIFIED.,.F.,.F.,(4,2,4),(0.223030667259691,0.241734353696197,
0.260285072590614),.UNSPECIFIED.);
#5417=B_SPLINE_CURVE_WITH_KNOTS('',3,(#64850,#64851,#64852,#64853,#64854,
#64855,#64856,#64857,#64858,#64859,#64860,#64861,#64862,#64863,#64864,#64865,
#64866,#64867,#64868,#64869,#64870,#64871,#64872,#64873,#64874,#64875,#64876,
#64877,#64878,#64879,#64880,#64881,#64882,#64883,#64884,#64885,#64886,#64887,
#64888,#64889,#64890,#64891,#64892,#64893,#64894,#64895,#64896,#64897,#64898,
#64899,#64900,#64901,#64902,#64903,#64904,#64905,#64906,#64907,#64908,#64909,
#64910),.UNSPECIFIED.,.F.,.F.,(4,3,3,3,3,3,3,3,3,3,3,3,3,3,3,3,3,3,3,3,
4),(0.,0.00795992543948654,0.0158204416141764,0.0168758198258157,0.0195772972159437,
0.0274588993006712,0.0354166538447632,0.0390209976709924,0.0469884348389282,
0.0505535087526213,0.0584240670042275,0.0663285883843903,0.0742861746185043,
0.0778995393740957,0.0842874233172874,0.0922711899963328,0.0975220154528215,
0.105525144757543,0.10781729367049,0.115774466403908,0.11811865411736),
 .UNSPECIFIED.);
#5418=B_SPLINE_CURVE_WITH_KNOTS('',3,(#64918,#64919,#64920,#64921,#64922,
#64923,#64924,#64925,#64926,#64927),.UNSPECIFIED.,.F.,.F.,(4,2,2,2,4),(0.0743659931772119,
0.0930945754988228,0.111742767843467,0.130288302686557,0.148746748488587),
 .UNSPECIFIED.);
#5419=B_SPLINE_CURVE_WITH_KNOTS('',3,(#64930,#64931,#64932,#64933,#64934,
#64935),.UNSPECIFIED.,.F.,.F.,(4,2,4),(0.223030667259691,0.241734353696197,
0.260285072590614),.UNSPECIFIED.);
#5420=B_SPLINE_CURVE_WITH_KNOTS('',3,(#64937,#64938,#64939,#64940,#64941,
#64942,#64943,#64944,#64945,#64946,#64947,#64948,#64949,#64950,#64951,#64952,
#64953,#64954,#64955,#64956,#64957,#64958,#64959,#64960,#64961,#64962,#64963,
#64964,#64965,#64966,#64967,#64968,#64969,#64970,#64971,#64972,#64973,#64974,
#64975,#64976,#64977,#64978,#64979,#64980,#64981,#64982,#64983,#64984,#64985,
#64986,#64987,#64988,#64989,#64990,#64991,#64992,#64993,#64994,#64995,#64996,
#64997),.UNSPECIFIED.,.F.,.F.,(4,3,3,3,3,3,3,3,3,3,3,3,3,3,3,3,3,3,3,3,
4),(0.,0.00795992543949775,0.0158204416141938,0.0168758198258168,0.0195772972159446,
0.0274588993006973,0.0354166538448255,0.039020997670994,0.0469884348389804,
0.0505535087526245,0.0584240670042325,0.0663285883843688,0.0742861746184431,
0.0778995393741076,0.0842874233172998,0.0922711899963224,0.097522015452835,
0.105525144757354,0.107817293670499,0.115774466404384,0.118118654117365),
 .UNSPECIFIED.);
#5421=B_SPLINE_CURVE_WITH_KNOTS('',3,(#65005,#65006,#65007,#65008,#65009,
#65010,#65011,#65012,#65013,#65014),.UNSPECIFIED.,.F.,.F.,(4,2,2,2,4),(0.0743659931772118,
0.0930945754988225,0.111742767843467,0.130288302686557,0.148746748488587),
 .UNSPECIFIED.);
#5422=B_SPLINE_CURVE_WITH_KNOTS('',3,(#65017,#65018,#65019,#65020,#65021,
#65022),.UNSPECIFIED.,.F.,.F.,(4,2,4),(0.223030667259692,0.241734353696198,
0.260285072590615),.UNSPECIFIED.);
#5423=B_SPLINE_CURVE_WITH_KNOTS('',3,(#65024,#65025,#65026,#65027,#65028,
#65029,#65030,#65031,#65032,#65033,#65034,#65035,#65036,#65037,#65038,#65039,
#65040,#65041,#65042,#65043,#65044,#65045,#65046,#65047,#65048,#65049,#65050,
#65051,#65052,#65053,#65054,#65055,#65056,#65057,#65058,#65059,#65060,#65061,
#65062,#65063,#65064,#65065,#65066,#65067,#65068,#65069,#65070,#65071,#65072,
#65073,#65074,#65075,#65076,#65077,#65078,#65079,#65080,#65081,#65082,#65083,
#65084),.UNSPECIFIED.,.F.,.F.,(4,3,3,3,3,3,3,3,3,3,3,3,3,3,3,3,3,3,3,3,
4),(0.,0.0079599254395225,0.0158204416142309,0.016875819825814,0.0195772972159418,
0.027458899300654,0.0354166538447342,0.0390209976709895,0.0469884348389785,
0.050553508752619,0.0584240670042285,0.0663285883843651,0.0742861746184472,
0.0778995393741052,0.0842874233172974,0.0922711899963051,0.0975220154528314,
0.105525144757553,0.107817293670496,0.115774466404379,0.118118654117369),
 .UNSPECIFIED.);
#5424=B_SPLINE_CURVE_WITH_KNOTS('',3,(#65089,#65090,#65091,#65092,#65093,
#65094),.UNSPECIFIED.,.F.,.F.,(4,2,4),(-0.0161375727826142,0.,0.000421605906895856),
 .UNSPECIFIED.);
#5425=B_SPLINE_CURVE_WITH_KNOTS('',3,(#65144,#65145,#65146,#65147,#65148,
#65149,#65150,#65151,#65152,#65153,#65154,#65155,#65156,#65157,#65158,#65159,
#65160,#65161,#65162,#65163,#65164,#65165,#65166,#65167,#65168,#65169,#65170,
#65171,#65172,#65173,#65174,#65175,#65176,#65177,#65178,#65179,#65180,#65181,
#65182,#65183,#65184,#65185,#65186,#65187,#65188,#65189,#65190,#65191,#65192,
#65193,#65194,#65195,#65196,#65197,#65198,#65199,#65200,#65201,#65202,#65203,
#65204),.UNSPECIFIED.,.F.,.F.,(4,3,3,3,3,3,3,3,3,3,3,3,3,3,3,3,3,3,3,3,
4),(0.,0.00788945390620875,0.0159107528337271,0.0198233466742035,0.0278090397101045,
0.0338830033915008,0.0395609471880769,0.047495504646808,0.05543216058732,
0.0591436409533866,0.0671079528129851,0.0676235550484156,0.0755926825994609,
0.0785910514609752,0.0865300392580439,0.0944439925210487,0.0979951919099191,
0.101302747945529,0.108060095589016,0.116004888439911,0.118137330218038),
 .UNSPECIFIED.);
#5426=B_SPLINE_CURVE_WITH_KNOTS('',3,(#65205,#65206,#65207,#65208),
 .UNSPECIFIED.,.F.,.F.,(4,4),(0.82916884759973,1.33025671401017),
 .UNSPECIFIED.);
#5427=B_SPLINE_CURVE_WITH_KNOTS('',3,(#65213,#65214,#65215,#65216,#65217,
#65218),.UNSPECIFIED.,.F.,.F.,(4,2,4),(0.0370807285215093,0.0556314474159263,
0.0743351338524322),.UNSPECIFIED.);
#5428=B_SPLINE_CURVE_WITH_KNOTS('',3,(#65227,#65228,#65229,#65230,#65231,
#65232,#65233,#65234,#65235,#65236),.UNSPECIFIED.,.F.,.F.,(4,2,2,2,4),(0.148746748488587,
0.167205194290616,0.185750729133706,0.204398921478351,0.223127503799962),
 .UNSPECIFIED.);
#5429=B_SPLINE_CURVE_WITH_KNOTS('',3,(#65265,#65266,#65267,#65268),
 .UNSPECIFIED.,.F.,.F.,(4,4),(0.829183372221167,1.33027123863146),
 .UNSPECIFIED.);
#5430=B_SPLINE_CURVE_WITH_KNOTS('',3,(#65305,#65306,#65307,#65308,#65309,
#65310,#65311,#65312,#65313,#65314,#65315,#65316,#65317,#65318,#65319,#65320,
#65321,#65322,#65323,#65324,#65325,#65326,#65327,#65328,#65329,#65330,#65331,
#65332,#65333,#65334,#65335,#65336,#65337,#65338,#65339,#65340,#65341,#65342,
#65343,#65344,#65345,#65346,#65347,#65348,#65349,#65350,#65351,#65352,#65353,
#65354,#65355,#65356,#65357,#65358,#65359,#65360,#65361,#65362,#65363,#65364,
#65365),.UNSPECIFIED.,.F.,.F.,(4,3,3,3,3,3,3,3,3,3,3,3,3,3,3,3,3,3,3,3,
4),(0.,0.00788945390620776,0.0159107528337215,0.019823346674202,0.0278090397100862,
0.0338830033914998,0.0395609471880765,0.0474955046467828,0.055432160587273,
0.0591436409533932,0.0671079528129883,0.0676235550484267,0.0755926825994682,
0.0785910514609908,0.0865300392580284,0.0944439925209911,0.0979951919099412,
0.101302747945553,0.108060095589036,0.116004888440633,0.118137330218056),
 .UNSPECIFIED.);
#5431=B_SPLINE_CURVE_WITH_KNOTS('',3,(#65366,#65367,#65368,#65369),
 .UNSPECIFIED.,.F.,.F.,(4,4),(0.829168847599735,1.33025671401018),
 .UNSPECIFIED.);
#5432=B_SPLINE_CURVE_WITH_KNOTS('',3,(#65383,#65384,#65385,#65386,#65387,
#65388,#65389,#65390,#65391,#65392),.UNSPECIFIED.,.F.,.F.,(4,2,2,2,4),(0.148746748488587,
0.167205194290616,0.185750729133706,0.204398921478351,0.223127503799961),
 .UNSPECIFIED.);
#5433=B_SPLINE_CURVE_WITH_KNOTS('',3,(#65398,#65399,#65400,#65401,#65402,
#65403),.UNSPECIFIED.,.F.,.F.,(4,2,4),(-0.200640408047776,-0.200218802140828,
-0.184081233349071),.UNSPECIFIED.);
#5434=B_SPLINE_CURVE_WITH_KNOTS('',3,(#65422,#65423,#65424,#65425),
 .UNSPECIFIED.,.F.,.F.,(4,4),(-0.08135049134023,-0.0743659931772121),
 .UNSPECIFIED.);
#5435=B_SPLINE_CURVE_WITH_KNOTS('',3,(#65434,#65435,#65436,#65437),
 .UNSPECIFIED.,.F.,.F.,(4,4),(-0.170732657218268,-0.156799509139685),
 .UNSPECIFIED.);
#5436=B_SPLINE_CURVE_WITH_KNOTS('',3,(#65439,#65440,#65441,#65442,#65443,
#65444),.UNSPECIFIED.,.F.,.F.,(4,2,4),(0.0250159248865165,0.262677835658091,
0.516689802275816),.UNSPECIFIED.);
#5437=B_SPLINE_CURVE_WITH_KNOTS('',3,(#65445,#65446,#65447,#65448),
 .UNSPECIFIED.,.F.,.F.,(4,4),(-0.35545892019756,-0.309416993782686),
 .UNSPECIFIED.);
#5438=B_SPLINE_CURVE_WITH_KNOTS('',3,(#65449,#65450,#65451,#65452,#65453,
#65454),.UNSPECIFIED.,.F.,.F.,(4,2,4),(0.0370807285215092,0.0556314474159263,
0.0743351338524322),.UNSPECIFIED.);
#5439=B_SPLINE_CURVE_WITH_KNOTS('',3,(#65466,#65467,#65468,#65469),
 .UNSPECIFIED.,.F.,.F.,(4,4),(-0.223127503799962,-0.216143005636944),
 .UNSPECIFIED.);
#5440=B_SPLINE_CURVE_WITH_KNOTS('',3,(#65481,#65482,#65483,#65484,#65485,
#65486,#65487,#65488,#65489,#65490,#65491,#65492),.UNSPECIFIED.,.F.,.F.,
(4,2,2,2,2,4),(0.,0.0146453155547523,0.0329425480524922,0.0585813427772626,
0.0866269082173564,0.08706621227491),.UNSPECIFIED.);
#5441=B_SPLINE_CURVE_WITH_KNOTS('',3,(#65494,#65495,#65496,#65497,#65498,
#65499,#65500,#65501,#65502,#65503,#65504,#65505),.UNSPECIFIED.,.F.,.F.,
(4,2,2,2,2,4),(-0.00044410187836752,0.,0.0380815409759577,0.0676748364251937,
0.0897163855604342,0.098171512873764),.UNSPECIFIED.);
#6178=LINE('',#63541,#7070);
#6179=LINE('',#63545,#7071);
#6180=LINE('',#63553,#7072);
#6181=LINE('',#63555,#7073);
#6182=LINE('',#63557,#7074);
#6183=LINE('',#63567,#7075);
#6184=LINE('',#63569,#7076);
#6185=LINE('',#63571,#7077);
#6186=LINE('',#63579,#7078);
#6187=LINE('',#63581,#7079);
#6188=LINE('',#63583,#7080);
#6189=LINE('',#63591,#7081);
#6190=LINE('',#63592,#7082);
#6191=LINE('',#63600,#7083);
#6192=LINE('',#63604,#7084);
#6193=LINE('',#63606,#7085);
#6194=LINE('',#63608,#7086);
#6195=LINE('',#63612,#7087);
#6196=LINE('',#63614,#7088);
#6197=LINE('',#63616,#7089);
#6198=LINE('',#63622,#7090);
#6199=LINE('',#63624,#7091);
#6200=LINE('',#63626,#7092);
#6201=LINE('',#63632,#7093);
#6202=LINE('',#63633,#7094);
#6203=LINE('',#63638,#7095);
#6204=LINE('',#63642,#7096);
#6205=LINE('',#63644,#7097);
#6206=LINE('',#63645,#7098);
#6207=LINE('',#63653,#7099);
#6208=LINE('',#63657,#7100);
#6209=LINE('',#63659,#7101);
#6210=LINE('',#63660,#7102);
#6211=LINE('',#63668,#7103);
#6212=LINE('',#63672,#7104);
#6213=LINE('',#63674,#7105);
#6214=LINE('',#63675,#7106);
#6215=LINE('',#63696,#7107);
#6216=LINE('',#63699,#7108);
#6217=LINE('',#63708,#7109);
#6218=LINE('',#63711,#7110);
#6219=LINE('',#63786,#7111);
#6220=LINE('',#63793,#7112);
#6221=LINE('',#63794,#7113);
#6222=LINE('',#63813,#7114);
#6223=LINE('',#63829,#7115);
#6224=LINE('',#63833,#7116);
#6225=LINE('',#63837,#7117);
#6226=LINE('',#63841,#7118);
#6227=LINE('',#63845,#7119);
#6228=LINE('',#63849,#7120);
#6229=LINE('',#63853,#7121);
#6230=LINE('',#63856,#7122);
#6231=LINE('',#63864,#7123);
#6232=LINE('',#63959,#7124);
#6233=LINE('',#63962,#7125);
#6234=LINE('',#64073,#7126);
#6235=LINE('',#64075,#7127);
#6236=LINE('',#64078,#7128);
#6237=LINE('',#64080,#7129);
#6238=LINE('',#64087,#7130);
#6239=LINE('',#64110,#7131);
#6240=LINE('',#64120,#7132);
#6241=LINE('',#64134,#7133);
#6242=LINE('',#64137,#7134);
#6243=LINE('',#64139,#7135);
#6244=LINE('',#64200,#7136);
#6245=LINE('',#64222,#7137);
#6246=LINE('',#64224,#7138);
#6247=LINE('',#64230,#7139);
#6248=LINE('',#64233,#7140);
#6249=LINE('',#64237,#7141);
#6250=LINE('',#64241,#7142);
#6251=LINE('',#64268,#7143);
#6252=LINE('',#64271,#7144);
#6253=LINE('',#64316,#7145);
#6254=LINE('',#64330,#7146);
#6255=LINE('',#64354,#7147);
#6256=LINE('',#64369,#7148);
#6257=LINE('',#64371,#7149);
#6258=LINE('',#64374,#7150);
#6259=LINE('',#64376,#7151);
#6260=LINE('',#64379,#7152);
#6261=LINE('',#64381,#7153);
#6262=LINE('',#64384,#7154);
#6263=LINE('',#64388,#7155);
#6264=LINE('',#64391,#7156);
#6265=LINE('',#64393,#7157);
#6266=LINE('',#64397,#7158);
#6267=LINE('',#64400,#7159);
#6268=LINE('',#64403,#7160);
#6269=LINE('',#64405,#7161);
#6270=LINE('',#64409,#7162);
#6271=LINE('',#64449,#7163);
#6272=LINE('',#64451,#7164);
#6273=LINE('',#64452,#7165);
#6274=LINE('',#64455,#7166);
#6275=LINE('',#64495,#7167);
#6276=LINE('',#64497,#7168);
#6277=LINE('',#64498,#7169);
#6278=LINE('',#64540,#7170);
#6279=LINE('',#64563,#7171);
#6280=LINE('',#64566,#7172);
#6281=LINE('',#64569,#7173);
#6282=LINE('',#64594,#7174);
#6283=LINE('',#64601,#7175);
#6284=LINE('',#64605,#7176);
#6285=LINE('',#64616,#7177);
#6286=LINE('',#64623,#7178);
#6287=LINE('',#64637,#7179);
#6288=LINE('',#64653,#7180);
#6289=LINE('',#64661,#7181);
#6290=LINE('',#64663,#7182);
#6291=LINE('',#64738,#7183);
#6292=LINE('',#64750,#7184);
#6293=LINE('',#64773,#7185);
#6294=LINE('',#64774,#7186);
#6295=LINE('',#64789,#7187);
#6296=LINE('',#64826,#7188);
#6297=LINE('',#64829,#7189);
#6298=LINE('',#64842,#7190);
#6299=LINE('',#64911,#7191);
#6300=LINE('',#64913,#7192);
#6301=LINE('',#64916,#7193);
#6302=LINE('',#64929,#7194);
#6303=LINE('',#64998,#7195);
#6304=LINE('',#65000,#7196);
#6305=LINE('',#65003,#7197);
#6306=LINE('',#65016,#7198);
#6307=LINE('',#65085,#7199);
#6308=LINE('',#65096,#7200);
#6309=LINE('',#65100,#7201);
#6310=LINE('',#65110,#7202);
#6311=LINE('',#65111,#7203);
#6312=LINE('',#65210,#7204);
#6313=LINE('',#65222,#7205);
#6314=LINE('',#65371,#7206);
#6315=LINE('',#65375,#7207);
#6316=LINE('',#65379,#7208);
#6317=LINE('',#65407,#7209);
#6318=LINE('',#65412,#7210);
#6319=LINE('',#65413,#7211);
#6320=LINE('',#65415,#7212);
#6321=LINE('',#65418,#7213);
#6322=LINE('',#65420,#7214);
#6323=LINE('',#65426,#7215);
#6324=LINE('',#65430,#7216);
#6325=LINE('',#65456,#7217);
#6326=LINE('',#65461,#7218);
#6327=LINE('',#65464,#7219);
#6328=LINE('',#65471,#7220);
#6329=LINE('',#65472,#7221);
#6330=LINE('',#65474,#7222);
#6331=LINE('',#65476,#7223);
#6332=LINE('',#65478,#7224);
#6333=LINE('',#65511,#7225);
#7070=VECTOR('',#26957,9.);
#7071=VECTOR('',#26960,10.);
#7072=VECTOR('',#26967,10.);
#7073=VECTOR('',#26968,10.);
#7074=VECTOR('',#26969,10.);
#7075=VECTOR('',#26978,10.);
#7076=VECTOR('',#26979,10.);
#7077=VECTOR('',#26980,10.);
#7078=VECTOR('',#26987,10.);
#7079=VECTOR('',#26988,10.);
#7080=VECTOR('',#26989,10.);
#7081=VECTOR('',#26996,10.);
#7082=VECTOR('',#26997,10.);
#7083=VECTOR('',#27006,10.);
#7084=VECTOR('',#27009,10.);
#7085=VECTOR('',#27010,10.);
#7086=VECTOR('',#27011,10.);
#7087=VECTOR('',#27014,10.);
#7088=VECTOR('',#27015,10.);
#7089=VECTOR('',#27016,10.);
#7090=VECTOR('',#27021,10.);
#7091=VECTOR('',#27022,10.);
#7092=VECTOR('',#27023,10.);
#7093=VECTOR('',#27028,10.);
#7094=VECTOR('',#27029,10.);
#7095=VECTOR('',#27034,10.);
#7096=VECTOR('',#27039,10.);
#7097=VECTOR('',#27040,10.);
#7098=VECTOR('',#27041,10.);
#7099=VECTOR('',#27052,10.);
#7100=VECTOR('',#27057,10.);
#7101=VECTOR('',#27058,10.);
#7102=VECTOR('',#27059,10.);
#7103=VECTOR('',#27070,10.);
#7104=VECTOR('',#27075,10.);
#7105=VECTOR('',#27076,10.);
#7106=VECTOR('',#27077,10.);
#7107=VECTOR('',#27104,10.);
#7108=VECTOR('',#27107,10.);
#7109=VECTOR('',#27120,10.);
#7110=VECTOR('',#27123,10.);
#7111=VECTOR('',#27134,10.);
#7112=VECTOR('',#27135,10.);
#7113=VECTOR('',#27136,10.);
#7114=VECTOR('',#27139,10.);
#7115=VECTOR('',#27162,21.);
#7116=VECTOR('',#27165,10.);
#7117=VECTOR('',#27168,10.);
#7118=VECTOR('',#27171,10.);
#7119=VECTOR('',#27174,10.);
#7120=VECTOR('',#27177,10.);
#7121=VECTOR('',#27180,10.);
#7122=VECTOR('',#27183,10.);
#7123=VECTOR('',#27192,10.);
#7124=VECTOR('',#27233,10.);
#7125=VECTOR('',#27236,10.);
#7126=VECTOR('',#27277,10.);
#7127=VECTOR('',#27280,10.);
#7128=VECTOR('',#27283,10.);
#7129=VECTOR('',#27284,10.);
#7130=VECTOR('',#27287,10.);
#7131=VECTOR('',#27298,10.);
#7132=VECTOR('',#27313,10.);
#7133=VECTOR('',#27314,10.);
#7134=VECTOR('',#27317,10.);
#7135=VECTOR('',#27318,10.);
#7136=VECTOR('',#27335,10.);
#7137=VECTOR('',#27346,10.);
#7138=VECTOR('',#27347,10.);
#7139=VECTOR('',#27348,10.);
#7140=VECTOR('',#27351,10.);
#7141=VECTOR('',#27356,10.);
#7142=VECTOR('',#27361,10.);
#7143=VECTOR('',#27378,10.);
#7144=VECTOR('',#27381,10.);
#7145=VECTOR('',#27394,10.);
#7146=VECTOR('',#27395,10.);
#7147=VECTOR('',#27406,10.);
#7148=VECTOR('',#27409,10.);
#7149=VECTOR('',#27410,10.);
#7150=VECTOR('',#27413,10.);
#7151=VECTOR('',#27414,10.);
#7152=VECTOR('',#27417,10.);
#7153=VECTOR('',#27418,18.5);
#7154=VECTOR('',#27421,10.);
#7155=VECTOR('',#27426,10.);
#7156=VECTOR('',#27429,10.);
#7157=VECTOR('',#27430,10.);
#7158=VECTOR('',#27433,10.);
#7159=VECTOR('',#27436,10.);
#7160=VECTOR('',#27439,10.);
#7161=VECTOR('',#27440,10.);
#7162=VECTOR('',#27445,10.);
#7163=VECTOR('',#27452,10.);
#7164=VECTOR('',#27453,10.);
#7165=VECTOR('',#27454,10.);
#7166=VECTOR('',#27457,10.);
#7167=VECTOR('',#27464,10.);
#7168=VECTOR('',#27465,10.);
#7169=VECTOR('',#27466,10.);
#7170=VECTOR('',#27483,10.);
#7171=VECTOR('',#27496,10.);
#7172=VECTOR('',#27499,10.);
#7173=VECTOR('',#27502,10.);
#7174=VECTOR('',#27509,10.);
#7175=VECTOR('',#27520,10.);
#7176=VECTOR('',#27525,10.);
#7177=VECTOR('',#27546,10.);
#7178=VECTOR('',#27555,10.);
#7179=VECTOR('',#27558,10.);
#7180=VECTOR('',#27563,10.);
#7181=VECTOR('',#27566,10.);
#7182=VECTOR('',#27567,10.);
#7183=VECTOR('',#27568,10.);
#7184=VECTOR('',#27569,10.);
#7185=VECTOR('',#27576,10.);
#7186=VECTOR('',#27577,10.);
#7187=VECTOR('',#27590,20.6);
#7188=VECTOR('',#27599,10.);
#7189=VECTOR('',#27602,10.);
#7190=VECTOR('',#27603,10.);
#7191=VECTOR('',#27604,10.);
#7192=VECTOR('',#27607,10.);
#7193=VECTOR('',#27610,10.);
#7194=VECTOR('',#27611,10.);
#7195=VECTOR('',#27612,10.);
#7196=VECTOR('',#27615,10.);
#7197=VECTOR('',#27618,10.);
#7198=VECTOR('',#27619,10.);
#7199=VECTOR('',#27620,10.);
#7200=VECTOR('',#27623,10.);
#7201=VECTOR('',#27626,10.);
#7202=VECTOR('',#27643,10.);
#7203=VECTOR('',#27644,10.);
#7204=VECTOR('',#27653,10.);
#7205=VECTOR('',#27660,10.);
#7206=VECTOR('',#27683,10.);
#7207=VECTOR('',#27686,10.);
#7208=VECTOR('',#27689,10.);
#7209=VECTOR('',#27702,10.);
#7210=VECTOR('',#27711,10.);
#7211=VECTOR('',#27712,10.);
#7212=VECTOR('',#27715,10.);
#7213=VECTOR('',#27718,10.);
#7214=VECTOR('',#27719,10.);
#7215=VECTOR('',#27720,10.);
#7216=VECTOR('',#27723,10.);
#7217=VECTOR('',#27730,10.);
#7218=VECTOR('',#27735,10.);
#7219=VECTOR('',#27738,10.);
#7220=VECTOR('',#27739,10.);
#7221=VECTOR('',#27740,10.);
#7222=VECTOR('',#27743,10.);
#7223=VECTOR('',#27746,10.);
#7224=VECTOR('',#27749,10.);
#7225=VECTOR('',#27766,10.);
#8859=VERTEX_POINT('',#63529);
#8860=VERTEX_POINT('',#63531);
#8861=VERTEX_POINT('',#63533);
#8862=VERTEX_POINT('',#63537);
#8863=VERTEX_POINT('',#63538);
#8864=VERTEX_POINT('',#63543);
#8865=VERTEX_POINT('',#63544);
#8866=VERTEX_POINT('',#63546);
#8867=VERTEX_POINT('',#63548);
#8868=VERTEX_POINT('',#63550);
#8869=VERTEX_POINT('',#63552);
#8870=VERTEX_POINT('',#63554);
#8871=VERTEX_POINT('',#63556);
#8872=VERTEX_POINT('',#63558);
#8873=VERTEX_POINT('',#63560);
#8874=VERTEX_POINT('',#63562);
#8875=VERTEX_POINT('',#63564);
#8876=VERTEX_POINT('',#63566);
#8877=VERTEX_POINT('',#63568);
#8878=VERTEX_POINT('',#63570);
#8879=VERTEX_POINT('',#63572);
#8880=VERTEX_POINT('',#63574);
#8881=VERTEX_POINT('',#63576);
#8882=VERTEX_POINT('',#63578);
#8883=VERTEX_POINT('',#63580);
#8884=VERTEX_POINT('',#63582);
#8885=VERTEX_POINT('',#63584);
#8886=VERTEX_POINT('',#63586);
#8887=VERTEX_POINT('',#63588);
#8888=VERTEX_POINT('',#63590);
#8889=VERTEX_POINT('',#63594);
#8890=VERTEX_POINT('',#63598);
#8891=VERTEX_POINT('',#63599);
#8892=VERTEX_POINT('',#63601);
#8893=VERTEX_POINT('',#63603);
#8894=VERTEX_POINT('',#63605);
#8895=VERTEX_POINT('',#63607);
#8896=VERTEX_POINT('',#63609);
#8897=VERTEX_POINT('',#63611);
#8898=VERTEX_POINT('',#63613);
#8899=VERTEX_POINT('',#63615);
#8900=VERTEX_POINT('',#63617);
#8901=VERTEX_POINT('',#63619);
#8902=VERTEX_POINT('',#63621);
#8903=VERTEX_POINT('',#63623);
#8904=VERTEX_POINT('',#63625);
#8905=VERTEX_POINT('',#63627);
#8906=VERTEX_POINT('',#63629);
#8907=VERTEX_POINT('',#63631);
#8908=VERTEX_POINT('',#63635);
#8909=VERTEX_POINT('',#63637);
#8910=VERTEX_POINT('',#63641);
#8911=VERTEX_POINT('',#63643);
#8912=VERTEX_POINT('',#63650);
#8913=VERTEX_POINT('',#63652);
#8914=VERTEX_POINT('',#63656);
#8915=VERTEX_POINT('',#63658);
#8916=VERTEX_POINT('',#63665);
#8917=VERTEX_POINT('',#63667);
#8918=VERTEX_POINT('',#63671);
#8919=VERTEX_POINT('',#63673);
#8920=VERTEX_POINT('',#63680);
#8921=VERTEX_POINT('',#63681);
#8922=VERTEX_POINT('',#63683);
#8923=VERTEX_POINT('',#63685);
#8924=VERTEX_POINT('',#63689);
#8925=VERTEX_POINT('',#63693);
#8926=VERTEX_POINT('',#63695);
#8927=VERTEX_POINT('',#63697);
#8928=VERTEX_POINT('',#63701);
#8929=VERTEX_POINT('',#63707);
#8930=VERTEX_POINT('',#63709);
#8931=VERTEX_POINT('',#63736);
#8932=VERTEX_POINT('',#63741);
#8933=VERTEX_POINT('',#63748);
#8934=VERTEX_POINT('',#63778);
#8935=VERTEX_POINT('',#63785);
#8936=VERTEX_POINT('',#63787);
#8937=VERTEX_POINT('',#63792);
#8938=VERTEX_POINT('',#63796);
#8939=VERTEX_POINT('',#63797);
#8940=VERTEX_POINT('',#63812);
#8941=VERTEX_POINT('',#63821);
#8942=VERTEX_POINT('',#63825);
#8943=VERTEX_POINT('',#63826);
#8944=VERTEX_POINT('',#63828);
#8945=VERTEX_POINT('',#63830);
#8946=VERTEX_POINT('',#63832);
#8947=VERTEX_POINT('',#63834);
#8948=VERTEX_POINT('',#63836);
#8949=VERTEX_POINT('',#63838);
#8950=VERTEX_POINT('',#63840);
#8951=VERTEX_POINT('',#63842);
#8952=VERTEX_POINT('',#63844);
#8953=VERTEX_POINT('',#63846);
#8954=VERTEX_POINT('',#63848);
#8955=VERTEX_POINT('',#63850);
#8956=VERTEX_POINT('',#63852);
#8957=VERTEX_POINT('',#63854);
#8958=VERTEX_POINT('',#63860);
#8959=VERTEX_POINT('',#63861);
#8960=VERTEX_POINT('',#63863);
#8961=VERTEX_POINT('',#63881);
#8962=VERTEX_POINT('',#63885);
#8963=VERTEX_POINT('',#63886);
#8964=VERTEX_POINT('',#63888);
#8965=VERTEX_POINT('',#63924);
#8966=VERTEX_POINT('',#63928);
#8967=VERTEX_POINT('',#63935);
#8968=VERTEX_POINT('',#63939);
#8969=VERTEX_POINT('',#63956);
#8970=VERTEX_POINT('',#63958);
#8971=VERTEX_POINT('',#63960);
#8972=VERTEX_POINT('',#63964);
#8973=VERTEX_POINT('',#63965);
#8974=VERTEX_POINT('',#63967);
#8975=VERTEX_POINT('',#63971);
#8976=VERTEX_POINT('',#63973);
#8977=VERTEX_POINT('',#63977);
#8978=VERTEX_POINT('',#63981);
#8979=VERTEX_POINT('',#63985);
#8980=VERTEX_POINT('',#63986);
#8981=VERTEX_POINT('',#63988);
#8982=VERTEX_POINT('',#64056);
#8983=VERTEX_POINT('',#64071);
#8984=VERTEX_POINT('',#64077);
#8985=VERTEX_POINT('',#64079);
#8986=VERTEX_POINT('',#64086);
#8987=VERTEX_POINT('',#64090);
#8988=VERTEX_POINT('',#64107);
#8989=VERTEX_POINT('',#64109);
#8990=VERTEX_POINT('',#64115);
#8991=VERTEX_POINT('',#64119);
#8992=VERTEX_POINT('',#64121);
#8993=VERTEX_POINT('',#64136);
#8994=VERTEX_POINT('',#64138);
#8995=VERTEX_POINT('',#64145);
#8996=VERTEX_POINT('',#64164);
#8997=VERTEX_POINT('',#64191);
#8998=VERTEX_POINT('',#64199);
#8999=VERTEX_POINT('',#64201);
#9000=VERTEX_POINT('',#64221);
#9001=VERTEX_POINT('',#64223);
#9002=VERTEX_POINT('',#64225);
#9003=VERTEX_POINT('',#64232);
#9004=VERTEX_POINT('',#64236);
#9005=VERTEX_POINT('',#64240);
#9006=VERTEX_POINT('',#64244);
#9007=VERTEX_POINT('',#64248);
#9008=VERTEX_POINT('',#64265);
#9009=VERTEX_POINT('',#64267);
#9010=VERTEX_POINT('',#64269);
#9011=VERTEX_POINT('',#64273);
#9012=VERTEX_POINT('',#64274);
#9013=VERTEX_POINT('',#64287);
#9014=VERTEX_POINT('',#64289);
#9015=VERTEX_POINT('',#64311);
#9016=VERTEX_POINT('',#64315);
#9017=VERTEX_POINT('',#64317);
#9018=VERTEX_POINT('',#64332);
#9019=VERTEX_POINT('',#64353);
#9020=VERTEX_POINT('',#64368);
#9021=VERTEX_POINT('',#64370);
#9022=VERTEX_POINT('',#64372);
#9023=VERTEX_POINT('',#64375);
#9024=VERTEX_POINT('',#64377);
#9025=VERTEX_POINT('',#64380);
#9026=VERTEX_POINT('',#64382);
#9027=VERTEX_POINT('',#64387);
#9028=VERTEX_POINT('',#64389);
#9029=VERTEX_POINT('',#64392);
#9030=VERTEX_POINT('',#64394);
#9031=VERTEX_POINT('',#64396);
#9032=VERTEX_POINT('',#64399);
#9033=VERTEX_POINT('',#64401);
#9034=VERTEX_POINT('',#64404);
#9035=VERTEX_POINT('',#64408);
#9036=VERTEX_POINT('',#64423);
#9037=VERTEX_POINT('',#64436);
#9038=VERTEX_POINT('',#64441);
#9039=VERTEX_POINT('',#64448);
#9040=VERTEX_POINT('',#64450);
#9041=VERTEX_POINT('',#64454);
#9042=VERTEX_POINT('',#64469);
#9043=VERTEX_POINT('',#64482);
#9044=VERTEX_POINT('',#64487);
#9045=VERTEX_POINT('',#64494);
#9046=VERTEX_POINT('',#64496);
#9047=VERTEX_POINT('',#64513);
#9048=VERTEX_POINT('',#64515);
#9049=VERTEX_POINT('',#64517);
#9050=VERTEX_POINT('',#64535);
#9051=VERTEX_POINT('',#64539);
#9052=VERTEX_POINT('',#64565);
#9053=VERTEX_POINT('',#64567);
#9054=VERTEX_POINT('',#64600);
#9055=VERTEX_POINT('',#64604);
#9056=VERTEX_POINT('',#64619);
#9057=VERTEX_POINT('',#64621);
#9058=VERTEX_POINT('',#64640);
#9059=VERTEX_POINT('',#64655);
#9060=VERTEX_POINT('',#64660);
#9061=VERTEX_POINT('',#64662);
#9062=VERTEX_POINT('',#64664);
#9063=VERTEX_POINT('',#64726);
#9064=VERTEX_POINT('',#64730);
#9065=VERTEX_POINT('',#64737);
#9066=VERTEX_POINT('',#64739);
#9067=VERTEX_POINT('',#64752);
#9068=VERTEX_POINT('',#64753);
#9069=VERTEX_POINT('',#64772);
#9070=VERTEX_POINT('',#64776);
#9071=VERTEX_POINT('',#64777);
#9072=VERTEX_POINT('',#64782);
#9073=VERTEX_POINT('',#64783);
#9074=VERTEX_POINT('',#64787);
#9075=VERTEX_POINT('',#64790);
#9076=VERTEX_POINT('',#64792);
#9077=VERTEX_POINT('',#64796);
#9078=VERTEX_POINT('',#64801);
#9079=VERTEX_POINT('',#64806);
#9080=VERTEX_POINT('',#64811);
#9081=VERTEX_POINT('',#64815);
#9082=VERTEX_POINT('',#64817);
#9083=VERTEX_POINT('',#64828);
#9084=VERTEX_POINT('',#64830);
#9085=VERTEX_POINT('',#64841);
#9086=VERTEX_POINT('',#64849);
#9087=VERTEX_POINT('',#64915);
#9088=VERTEX_POINT('',#64917);
#9089=VERTEX_POINT('',#64928);
#9090=VERTEX_POINT('',#64936);
#9091=VERTEX_POINT('',#65002);
#9092=VERTEX_POINT('',#65004);
#9093=VERTEX_POINT('',#65015);
#9094=VERTEX_POINT('',#65023);
#9095=VERTEX_POINT('',#65087);
#9096=VERTEX_POINT('',#65088);
#9097=VERTEX_POINT('',#65095);
#9098=VERTEX_POINT('',#65097);
#9099=VERTEX_POINT('',#65099);
#9100=VERTEX_POINT('',#65103);
#9101=VERTEX_POINT('',#65143);
#9102=VERTEX_POINT('',#65212);
#9103=VERTEX_POINT('',#65221);
#9104=VERTEX_POINT('',#65225);
#9105=VERTEX_POINT('',#65304);
#9106=VERTEX_POINT('',#65373);
#9107=VERTEX_POINT('',#65374);
#9108=VERTEX_POINT('',#65376);
#9109=VERTEX_POINT('',#65378);
#9110=VERTEX_POINT('',#65382);
#9111=VERTEX_POINT('',#65393);
#9112=VERTEX_POINT('',#65397);
#9113=VERTEX_POINT('',#65404);
#9114=VERTEX_POINT('',#65406);
#9115=VERTEX_POINT('',#65417);
#9116=VERTEX_POINT('',#65419);
#9117=VERTEX_POINT('',#65421);
#9118=VERTEX_POINT('',#65427);
#9119=VERTEX_POINT('',#65429);
#9120=VERTEX_POINT('',#65433);
#9121=VERTEX_POINT('',#65438);
#9122=VERTEX_POINT('',#65458);
#9123=VERTEX_POINT('',#65460);
#9124=VERTEX_POINT('',#65463);
#9125=VERTEX_POINT('',#65465);
#9126=VERTEX_POINT('',#65470);
#11753=EDGE_CURVE('',#8859,#8859,#4483,.T.);
#11754=EDGE_CURVE('',#8859,#8860,#4484,.T.);
#11755=EDGE_CURVE('',#8860,#8861,#4485,.T.);
#11756=EDGE_CURVE('',#8861,#8860,#4486,.T.);
#11757=EDGE_CURVE('',#8862,#8863,#4487,.T.);
#11758=EDGE_CURVE('',#8863,#8862,#4488,.T.);
#11759=EDGE_CURVE('',#8863,#8861,#6178,.T.);
#11760=EDGE_CURVE('',#8864,#8865,#6179,.T.);
#11761=EDGE_CURVE('',#8866,#8865,#4489,.F.);
#11762=EDGE_CURVE('',#8867,#8866,#4490,.T.);
#11763=EDGE_CURVE('',#8868,#8867,#4491,.F.);
#11764=EDGE_CURVE('',#8868,#8869,#6180,.T.);
#11765=EDGE_CURVE('',#8870,#8869,#6181,.T.);
#11766=EDGE_CURVE('',#8870,#8871,#6182,.T.);
#11767=EDGE_CURVE('',#8872,#8871,#4492,.F.);
#11768=EDGE_CURVE('',#8873,#8872,#4493,.T.);
#11769=EDGE_CURVE('',#8874,#8873,#4494,.T.);
#11770=EDGE_CURVE('',#8875,#8874,#4495,.F.);
#11771=EDGE_CURVE('',#8875,#8876,#6183,.T.);
#11772=EDGE_CURVE('',#8877,#8876,#6184,.T.);
#11773=EDGE_CURVE('',#8877,#8878,#6185,.T.);
#11774=EDGE_CURVE('',#8879,#8878,#4496,.F.);
#11775=EDGE_CURVE('',#8880,#8879,#4497,.T.);
#11776=EDGE_CURVE('',#8881,#8880,#4498,.F.);
#11777=EDGE_CURVE('',#8881,#8882,#6186,.T.);
#11778=EDGE_CURVE('',#8883,#8882,#6187,.T.);
#11779=EDGE_CURVE('',#8883,#8884,#6188,.T.);
#11780=EDGE_CURVE('',#8885,#8884,#4499,.F.);
#11781=EDGE_CURVE('',#8886,#8885,#4500,.T.);
#11782=EDGE_CURVE('',#8887,#8886,#4501,.F.);
#11783=EDGE_CURVE('',#8887,#8888,#6189,.T.);
#11784=EDGE_CURVE('',#8864,#8888,#6190,.T.);
#11785=EDGE_CURVE('',#8862,#8889,#4502,.T.);
#11786=EDGE_CURVE('',#8889,#8889,#4503,.T.);
#11787=EDGE_CURVE('',#8890,#8891,#6191,.T.);
#11788=EDGE_CURVE('',#8891,#8892,#4504,.T.);
#11789=EDGE_CURVE('',#8892,#8893,#6192,.T.);
#11790=EDGE_CURVE('',#8894,#8893,#6193,.T.);
#11791=EDGE_CURVE('',#8894,#8895,#6194,.T.);
#11792=EDGE_CURVE('',#8895,#8896,#4505,.T.);
#11793=EDGE_CURVE('',#8896,#8897,#6195,.T.);
#11794=EDGE_CURVE('',#8898,#8897,#6196,.T.);
#11795=EDGE_CURVE('',#8898,#8899,#6197,.T.);
#11796=EDGE_CURVE('',#8899,#8900,#4506,.T.);
#11797=EDGE_CURVE('',#8901,#8900,#4507,.F.);
#11798=EDGE_CURVE('',#8901,#8902,#6198,.T.);
#11799=EDGE_CURVE('',#8903,#8902,#6199,.T.);
#11800=EDGE_CURVE('',#8903,#8904,#6200,.T.);
#11801=EDGE_CURVE('',#8905,#8904,#4508,.F.);
#11802=EDGE_CURVE('',#8905,#8906,#4509,.T.);
#11803=EDGE_CURVE('',#8906,#8907,#6201,.T.);
#11804=EDGE_CURVE('',#8890,#8907,#6202,.T.);
#11805=EDGE_CURVE('',#8888,#8908,#4510,.F.);
#11806=EDGE_CURVE('',#8908,#8909,#6203,.T.);
#11807=EDGE_CURVE('',#8909,#8864,#4511,.F.);
#11808=EDGE_CURVE('',#8908,#8910,#6204,.T.);
#11809=EDGE_CURVE('',#8911,#8910,#6205,.T.);
#11810=EDGE_CURVE('',#8909,#8911,#6206,.T.);
#11811=EDGE_CURVE('',#8907,#8911,#4512,.F.);
#11812=EDGE_CURVE('',#8910,#8890,#4513,.F.);
#11813=EDGE_CURVE('',#8882,#8912,#4514,.F.);
#11814=EDGE_CURVE('',#8912,#8913,#6207,.T.);
#11815=EDGE_CURVE('',#8913,#8883,#4515,.F.);
#11816=EDGE_CURVE('',#8912,#8914,#6208,.T.);
#11817=EDGE_CURVE('',#8915,#8914,#6209,.T.);
#11818=EDGE_CURVE('',#8913,#8915,#6210,.T.);
#11819=EDGE_CURVE('',#8893,#8915,#4516,.F.);
#11820=EDGE_CURVE('',#8914,#8894,#4517,.F.);
#11821=EDGE_CURVE('',#8876,#8916,#4518,.F.);
#11822=EDGE_CURVE('',#8916,#8917,#6211,.T.);
#11823=EDGE_CURVE('',#8917,#8877,#4519,.F.);
#11824=EDGE_CURVE('',#8916,#8918,#6212,.T.);
#11825=EDGE_CURVE('',#8919,#8918,#6213,.T.);
#11826=EDGE_CURVE('',#8917,#8919,#6214,.T.);
#11827=EDGE_CURVE('',#8897,#8919,#4520,.F.);
#11828=EDGE_CURVE('',#8918,#8898,#4521,.F.);
#11829=EDGE_CURVE('',#8920,#8921,#4522,.T.);
#11830=EDGE_CURVE('',#8921,#8922,#4523,.T.);
#11831=EDGE_CURVE('',#8922,#8923,#4524,.T.);
#11832=EDGE_CURVE('',#8923,#8920,#4525,.T.);
#11833=EDGE_CURVE('',#8922,#8924,#4526,.T.);
#11834=EDGE_CURVE('',#8924,#8923,#4527,.T.);
#11835=EDGE_CURVE('',#8925,#8920,#4528,.T.);
#11836=EDGE_CURVE('',#8920,#8926,#6215,.T.);
#11837=EDGE_CURVE('',#8926,#8927,#4529,.T.);
#11838=EDGE_CURVE('',#8927,#8925,#6216,.T.);
#11839=EDGE_CURVE('',#8926,#8928,#4530,.T.);
#11840=EDGE_CURVE('',#8928,#8927,#4531,.T.);
#11841=EDGE_CURVE('',#8925,#8921,#4532,.T.);
#11842=EDGE_CURVE('',#8924,#8929,#6217,.T.);
#11843=EDGE_CURVE('',#8929,#8930,#4533,.T.);
#11844=EDGE_CURVE('',#8930,#8923,#6218,.T.);
#11845=EDGE_CURVE('',#8922,#8931,#5357,.T.);
#11846=EDGE_CURVE('',#8932,#8931,#4534,.T.);
#11847=EDGE_CURVE('',#8932,#8924,#5358,.T.);
#11848=EDGE_CURVE('',#8933,#8921,#5359,.T.);
#11849=EDGE_CURVE('',#8931,#8933,#4535,.T.);
#11850=EDGE_CURVE('',#8925,#8934,#5360,.T.);
#11851=EDGE_CURVE('',#8934,#8933,#4536,.T.);
#11852=EDGE_CURVE('',#8935,#8927,#6219,.T.);
#11853=EDGE_CURVE('',#8936,#8935,#5361,.T.);
#11854=EDGE_CURVE('',#8936,#8937,#6220,.T.);
#11855=EDGE_CURVE('',#8934,#8937,#6221,.T.);
#11856=EDGE_CURVE('',#8938,#8939,#5362,.T.);
#11857=EDGE_CURVE('',#8938,#8940,#6222,.T.);
#11858=EDGE_CURVE('',#8940,#8934,#4537,.T.);
#11859=EDGE_CURVE('',#8939,#8937,#4538,.T.);
#11860=EDGE_CURVE('',#8940,#8933,#4539,.T.);
#11861=EDGE_CURVE('',#8926,#8930,#4540,.T.);
#11862=EDGE_CURVE('',#8940,#8941,#4541,.T.);
#11863=EDGE_CURVE('',#8931,#8941,#4542,.T.);
#11864=EDGE_CURVE('',#8942,#8943,#4543,.T.);
#11865=EDGE_CURVE('',#8942,#8944,#6223,.T.);
#11866=EDGE_CURVE('',#8944,#8945,#4544,.T.);
#11867=EDGE_CURVE('',#8946,#8945,#6224,.T.);
#11868=EDGE_CURVE('',#8946,#8947,#4545,.T.);
#11869=EDGE_CURVE('',#8948,#8947,#6225,.T.);
#11870=EDGE_CURVE('',#8949,#8948,#4546,.T.);
#11871=EDGE_CURVE('',#8950,#8949,#6226,.T.);
#11872=EDGE_CURVE('',#8951,#8950,#4547,.T.);
#11873=EDGE_CURVE('',#8952,#8951,#6227,.T.);
#11874=EDGE_CURVE('',#8952,#8953,#4548,.T.);
#11875=EDGE_CURVE('',#8954,#8953,#6228,.T.);
#11876=EDGE_CURVE('',#8955,#8954,#4549,.T.);
#11877=EDGE_CURVE('',#8956,#8955,#6229,.T.);
#11878=EDGE_CURVE('',#8957,#8956,#4550,.T.);
#11879=EDGE_CURVE('',#8941,#8957,#6230,.T.);
#11880=EDGE_CURVE('',#8938,#8944,#4551,.T.);
#11881=EDGE_CURVE('',#8943,#8942,#4552,.T.);
#11882=EDGE_CURVE('',#8958,#8959,#4553,.F.);
#11883=EDGE_CURVE('',#8959,#8960,#6231,.T.);
#11884=EDGE_CURVE('',#8960,#8954,#4554,.T.);
#11885=EDGE_CURVE('',#8953,#8958,#5363,.F.);
#11886=EDGE_CURVE('',#8960,#8961,#4555,.T.);
#11887=EDGE_CURVE('',#8961,#8954,#4556,.T.);
#11888=EDGE_CURVE('',#8962,#8963,#4557,.T.);
#11889=EDGE_CURVE('',#8963,#8964,#4558,.T.);
#11890=EDGE_CURVE('',#8964,#8962,#4559,.T.);
#11891=EDGE_CURVE('',#8962,#8961,#5364,.T.);
#11892=EDGE_CURVE('',#8960,#8963,#5365,.T.);
#11893=EDGE_CURVE('',#8961,#8965,#4560,.T.);
#11894=EDGE_CURVE('',#8955,#8965,#4561,.T.);
#11895=EDGE_CURVE('',#8966,#8962,#4562,.T.);
#11896=EDGE_CURVE('',#8965,#8966,#5366,.T.);
#11897=EDGE_CURVE('',#8964,#8967,#4563,.T.);
#11898=EDGE_CURVE('',#8967,#8966,#4564,.T.);
#11899=EDGE_CURVE('',#8952,#8968,#5367,.F.);
#11900=EDGE_CURVE('',#8968,#8958,#4565,.T.);
#11901=EDGE_CURVE('',#8969,#8968,#4566,.F.);
#11902=EDGE_CURVE('',#8970,#8969,#6232,.T.);
#11903=EDGE_CURVE('',#8971,#8970,#4567,.T.);
#11904=EDGE_CURVE('',#8959,#8971,#6233,.T.);
#11905=EDGE_CURVE('',#8972,#8973,#4568,.T.);
#11906=EDGE_CURVE('',#8973,#8974,#4569,.T.);
#11907=EDGE_CURVE('',#8974,#8972,#4570,.T.);
#11908=EDGE_CURVE('',#8950,#8975,#4571,.T.);
#11909=EDGE_CURVE('',#8975,#8976,#4572,.T.);
#11910=EDGE_CURVE('',#8976,#8951,#4573,.T.);
#11911=EDGE_CURVE('',#8977,#8975,#4574,.T.);
#11912=EDGE_CURVE('',#8950,#8977,#4575,.T.);
#11913=EDGE_CURVE('',#8976,#8978,#4576,.T.);
#11914=EDGE_CURVE('',#8978,#8951,#4577,.T.);
#11915=EDGE_CURVE('',#8979,#8980,#4578,.T.);
#11916=EDGE_CURVE('',#8980,#8981,#4579,.T.);
#11917=EDGE_CURVE('',#8981,#8979,#4580,.T.);
#11918=EDGE_CURVE('',#8979,#8978,#5368,.T.);
#11919=EDGE_CURVE('',#8976,#8980,#5369,.T.);
#11920=EDGE_CURVE('',#8977,#8973,#5370,.T.);
#11921=EDGE_CURVE('',#8972,#8975,#5371,.T.);
#11922=EDGE_CURVE('',#8982,#8949,#5372,.F.);
#11923=EDGE_CURVE('',#8982,#8983,#4581,.F.);
#11924=EDGE_CURVE('',#8983,#8977,#6234,.T.);
#11925=EDGE_CURVE('',#8978,#8969,#6235,.T.);
#11926=EDGE_CURVE('',#8984,#8979,#6236,.T.);
#11927=EDGE_CURVE('',#8985,#8984,#6237,.T.);
#11928=EDGE_CURVE('',#8985,#8970,#5373,.T.);
#11929=EDGE_CURVE('',#8981,#8986,#6238,.T.);
#11930=EDGE_CURVE('',#8986,#8984,#4582,.F.);
#11931=EDGE_CURVE('',#8939,#8987,#4583,.T.);
#11932=EDGE_CURVE('',#8987,#8945,#5374,.F.);
#11933=EDGE_CURVE('',#8988,#8936,#4584,.T.);
#11934=EDGE_CURVE('',#8989,#8988,#6239,.T.);
#11935=EDGE_CURVE('',#8987,#8989,#4585,.F.);
#11936=EDGE_CURVE('',#8941,#8932,#4586,.T.);
#11937=EDGE_CURVE('',#8929,#8990,#4587,.T.);
#11938=EDGE_CURVE('',#8990,#8930,#4588,.T.);
#11939=EDGE_CURVE('',#8929,#8991,#6240,.T.);
#11940=EDGE_CURVE('',#8991,#8992,#5375,.T.);
#11941=EDGE_CURVE('',#8992,#8990,#6241,.T.);
#11942=EDGE_CURVE('',#8993,#8932,#6242,.T.);
#11943=EDGE_CURVE('',#8993,#8994,#6243,.T.);
#11944=EDGE_CURVE('',#8991,#8994,#5376,.T.);
#11945=EDGE_CURVE('',#8957,#8995,#5377,.T.);
#11946=EDGE_CURVE('',#8995,#8993,#4589,.T.);
#11947=EDGE_CURVE('',#8996,#8966,#4590,.T.);
#11948=EDGE_CURVE('',#8967,#8996,#4591,.T.);
#11949=EDGE_CURVE('',#8997,#8965,#4592,.T.);
#11950=EDGE_CURVE('',#8996,#8997,#5378,.T.);
#11951=EDGE_CURVE('',#8955,#8997,#4593,.T.);
#11952=EDGE_CURVE('',#8997,#8998,#6244,.T.);
#11953=EDGE_CURVE('',#8998,#8999,#4594,.T.);
#11954=EDGE_CURVE('',#8999,#8956,#5379,.T.);
#11955=EDGE_CURVE('',#8999,#8995,#4595,.T.);
#11956=EDGE_CURVE('',#9000,#8996,#6245,.T.);
#11957=EDGE_CURVE('',#9001,#9000,#6246,.T.);
#11958=EDGE_CURVE('',#9002,#9001,#5380,.T.);
#11959=EDGE_CURVE('',#9002,#8998,#6247,.T.);
#11960=EDGE_CURVE('',#8967,#9003,#6248,.T.);
#11961=EDGE_CURVE('',#9003,#9000,#4596,.T.);
#11962=EDGE_CURVE('',#9004,#8964,#6249,.T.);
#11963=EDGE_CURVE('',#9003,#9004,#4597,.T.);
#11964=EDGE_CURVE('',#8963,#9005,#6250,.T.);
#11965=EDGE_CURVE('',#9005,#9004,#4598,.T.);
#11966=EDGE_CURVE('',#9005,#9006,#4599,.T.);
#11967=EDGE_CURVE('',#9006,#9004,#4600,.T.);
#11968=EDGE_CURVE('',#8948,#9007,#5381,.F.);
#11969=EDGE_CURVE('',#9007,#8982,#4601,.T.);
#11970=EDGE_CURVE('',#9008,#9007,#4602,.F.);
#11971=EDGE_CURVE('',#9009,#9008,#6251,.T.);
#11972=EDGE_CURVE('',#9010,#9009,#4603,.T.);
#11973=EDGE_CURVE('',#8983,#9010,#6252,.T.);
#11974=EDGE_CURVE('',#9011,#9012,#5382,.T.);
#11975=EDGE_CURVE('',#9011,#9013,#4604,.T.);
#11976=EDGE_CURVE('',#9013,#9014,#5383,.F.);
#11977=EDGE_CURVE('',#9014,#9010,#5384,.F.);
#11978=EDGE_CURVE('',#9012,#9009,#5385,.T.);
#11979=EDGE_CURVE('',#9006,#9015,#4605,.T.);
#11980=EDGE_CURVE('',#9015,#9003,#4606,.T.);
#11981=EDGE_CURVE('',#9005,#9016,#6253,.T.);
#11982=EDGE_CURVE('',#9016,#9017,#5386,.T.);
#11983=EDGE_CURVE('',#9017,#9006,#6254,.T.);
#11984=EDGE_CURVE('',#9018,#8985,#5387,.T.);
#11985=EDGE_CURVE('',#9018,#9017,#4607,.T.);
#11986=EDGE_CURVE('',#9016,#8971,#5388,.T.);
#11987=EDGE_CURVE('',#9015,#9000,#4608,.T.);
#11988=EDGE_CURVE('',#9015,#9019,#6255,.T.);
#11989=EDGE_CURVE('',#9019,#9001,#5389,.T.);
#11990=EDGE_CURVE('',#8886,#9020,#6256,.T.);
#11991=EDGE_CURVE('',#8885,#9021,#6257,.T.);
#11992=EDGE_CURVE('',#9022,#9021,#4609,.T.);
#11993=EDGE_CURVE('',#8880,#9022,#6258,.T.);
#11994=EDGE_CURVE('',#8879,#9023,#6259,.T.);
#11995=EDGE_CURVE('',#9024,#9023,#4610,.T.);
#11996=EDGE_CURVE('',#8874,#9024,#6260,.T.);
#11997=EDGE_CURVE('',#8873,#9025,#6261,.T.);
#11998=EDGE_CURVE('',#9026,#9025,#4611,.T.);
#11999=EDGE_CURVE('',#8928,#9026,#6262,.T.);
#12000=EDGE_CURVE('',#8990,#8928,#4612,.T.);
#12001=EDGE_CURVE('',#9019,#8992,#4613,.T.);
#12002=EDGE_CURVE('',#9018,#9027,#6263,.T.);
#12003=EDGE_CURVE('',#9028,#9027,#4614,.T.);
#12004=EDGE_CURVE('',#9028,#9013,#6264,.T.);
#12005=EDGE_CURVE('',#9011,#9029,#6265,.T.);
#12006=EDGE_CURVE('',#9030,#9029,#4615,.T.);
#12007=EDGE_CURVE('',#9031,#9030,#6266,.T.);
#12008=EDGE_CURVE('',#9025,#9031,#4616,.T.);
#12009=EDGE_CURVE('',#9032,#8872,#6267,.T.);
#12010=EDGE_CURVE('',#9033,#9032,#4617,.T.);
#12011=EDGE_CURVE('',#8867,#9033,#6268,.T.);
#12012=EDGE_CURVE('',#8866,#9034,#6269,.T.);
#12013=EDGE_CURVE('',#9020,#9034,#4618,.T.);
#12014=EDGE_CURVE('',#9035,#8887,#6270,.T.);
#12015=EDGE_CURVE('',#9020,#9035,#5390,.T.);
#12016=EDGE_CURVE('',#9034,#9036,#5391,.F.);
#12017=EDGE_CURVE('',#9036,#9037,#5392,.F.);
#12018=EDGE_CURVE('',#9037,#9038,#4619,.T.);
#12019=EDGE_CURVE('',#9038,#9035,#5393,.T.);
#12020=EDGE_CURVE('',#9037,#9039,#6271,.T.);
#12021=EDGE_CURVE('',#9039,#9040,#6272,.T.);
#12022=EDGE_CURVE('',#9040,#9038,#6273,.T.);
#12023=EDGE_CURVE('',#9041,#8875,#6274,.T.);
#12024=EDGE_CURVE('',#9024,#9041,#5394,.T.);
#12025=EDGE_CURVE('',#9023,#9042,#5395,.F.);
#12026=EDGE_CURVE('',#9042,#9043,#5396,.F.);
#12027=EDGE_CURVE('',#9043,#9044,#4620,.T.);
#12028=EDGE_CURVE('',#9044,#9041,#5397,.T.);
#12029=EDGE_CURVE('',#9043,#9045,#6275,.T.);
#12030=EDGE_CURVE('',#9045,#9046,#6276,.T.);
#12031=EDGE_CURVE('',#9046,#9044,#6277,.T.);
#12032=EDGE_CURVE('',#9026,#8935,#5398,.T.);
#12033=EDGE_CURVE('',#9029,#9047,#4621,.T.);
#12034=EDGE_CURVE('',#9047,#9048,#4622,.T.);
#12035=EDGE_CURVE('',#9048,#9049,#5399,.T.);
#12036=EDGE_CURVE('',#9049,#9030,#5400,.T.);
#12037=EDGE_CURVE('',#9029,#9050,#4623,.T.);
#12038=EDGE_CURVE('',#9050,#9047,#4624,.T.);
#12039=EDGE_CURVE('',#9049,#9051,#6278,.T.);
#12040=EDGE_CURVE('',#9051,#9031,#5401,.T.);
#12041=EDGE_CURVE('',#9051,#8988,#5402,.T.);
#12042=EDGE_CURVE('',#8994,#9002,#4625,.T.);
#12043=EDGE_CURVE('',#9012,#9050,#6279,.T.);
#12044=EDGE_CURVE('',#9050,#9052,#6280,.T.);
#12045=EDGE_CURVE('',#9052,#9053,#4626,.T.);
#12046=EDGE_CURVE('',#9053,#9047,#6281,.T.);
#12047=EDGE_CURVE('',#8947,#9053,#5403,.T.);
#12048=EDGE_CURVE('',#9052,#8947,#4627,.T.);
#12049=EDGE_CURVE('',#9052,#9008,#6282,.T.);
#12050=EDGE_CURVE('',#8974,#8981,#4628,.T.);
#12051=EDGE_CURVE('',#8980,#8972,#4629,.T.);
#12052=EDGE_CURVE('',#9054,#8974,#6283,.T.);
#12053=EDGE_CURVE('',#8986,#9054,#4630,.T.);
#12054=EDGE_CURVE('',#8973,#9055,#6284,.T.);
#12055=EDGE_CURVE('',#9055,#9054,#4631,.F.);
#12056=EDGE_CURVE('',#9028,#9055,#4632,.F.);
#12057=EDGE_CURVE('',#9054,#9028,#4633,.F.);
#12058=EDGE_CURVE('',#9027,#8986,#4634,.F.);
#12059=EDGE_CURVE('',#8984,#9027,#4635,.F.);
#12060=EDGE_CURVE('',#9055,#9014,#6285,.T.);
#12061=EDGE_CURVE('',#9056,#9053,#4636,.T.);
#12062=EDGE_CURVE('',#9057,#9056,#4637,.T.);
#12063=EDGE_CURVE('',#9057,#9048,#6286,.T.);
#12064=EDGE_CURVE('',#9056,#8946,#5404,.T.);
#12065=EDGE_CURVE('',#8989,#9057,#6287,.T.);
#12066=EDGE_CURVE('',#9022,#9058,#5405,.F.);
#12067=EDGE_CURVE('',#9058,#8881,#6288,.T.);
#12068=EDGE_CURVE('',#9059,#9058,#5406,.F.);
#12069=EDGE_CURVE('',#9060,#9059,#6289,.T.);
#12070=EDGE_CURVE('',#9060,#9061,#6290,.T.);
#12071=EDGE_CURVE('',#9062,#9061,#5407,.F.);
#12072=EDGE_CURVE('',#9062,#9063,#828,.T.);
#12073=EDGE_CURVE('',#9063,#9064,#5408,.T.);
#12074=EDGE_CURVE('',#9065,#9064,#6291,.T.);
#12075=EDGE_CURVE('',#9066,#9065,#5409,.T.);
#12076=EDGE_CURVE('',#8895,#9066,#6292,.T.);
#12077=EDGE_CURVE('',#9067,#9068,#5410,.F.);
#12078=EDGE_CURVE('',#9068,#9059,#4638,.T.);
#12079=EDGE_CURVE('',#9021,#9067,#5411,.F.);
#12080=EDGE_CURVE('',#9068,#9069,#6293,.T.);
#12081=EDGE_CURVE('',#9069,#9060,#6294,.T.);
#12082=EDGE_CURVE('',#9070,#9071,#4639,.T.);
#12083=EDGE_CURVE('',#9071,#9070,#4640,.T.);
#12084=EDGE_CURVE('',#9070,#8943,#4641,.T.);
#12085=EDGE_CURVE('',#9072,#9073,#829,.T.);
#12086=EDGE_CURVE('',#9074,#9072,#4642,.T.);
#12087=EDGE_CURVE('',#9074,#9071,#6295,.T.);
#12088=EDGE_CURVE('',#9075,#9074,#4643,.T.);
#12089=EDGE_CURVE('',#9076,#9075,#830,.T.);
#12090=EDGE_CURVE('',#9077,#9076,#5412,.T.);
#12091=EDGE_CURVE('',#9078,#9077,#831,.T.);
#12092=EDGE_CURVE('',#9063,#9078,#4644,.T.);
#12093=EDGE_CURVE('',#9079,#9062,#5413,.T.);
#12094=EDGE_CURVE('',#9080,#9079,#832,.T.);
#12095=EDGE_CURVE('',#9081,#9080,#4645,.T.);
#12096=EDGE_CURVE('',#9082,#9081,#833,.T.);
#12097=EDGE_CURVE('',#9073,#9082,#5414,.T.);
#12098=EDGE_CURVE('',#8878,#9042,#6296,.T.);
#12099=EDGE_CURVE('',#9083,#8896,#6297,.T.);
#12100=EDGE_CURVE('',#9084,#9083,#5415,.T.);
#12101=EDGE_CURVE('',#9084,#9085,#6298,.T.);
#12102=EDGE_CURVE('',#9085,#9078,#5416,.T.);
#12103=EDGE_CURVE('',#9077,#9086,#5417,.T.);
#12104=EDGE_CURVE('',#9045,#9086,#6299,.T.);
#12105=EDGE_CURVE('',#8884,#9067,#6300,.T.);
#12106=EDGE_CURVE('',#9087,#8892,#6301,.T.);
#12107=EDGE_CURVE('',#9088,#9087,#5418,.T.);
#12108=EDGE_CURVE('',#9088,#9089,#6302,.T.);
#12109=EDGE_CURVE('',#9089,#9080,#5419,.T.);
#12110=EDGE_CURVE('',#9079,#9090,#5420,.T.);
#12111=EDGE_CURVE('',#9069,#9090,#6303,.T.);
#12112=EDGE_CURVE('',#8865,#9036,#6304,.T.);
#12113=EDGE_CURVE('',#9091,#8906,#6305,.T.);
#12114=EDGE_CURVE('',#9092,#9091,#5421,.T.);
#12115=EDGE_CURVE('',#9092,#9093,#6306,.T.);
#12116=EDGE_CURVE('',#9093,#9072,#5422,.T.);
#12117=EDGE_CURVE('',#9073,#9094,#5423,.T.);
#12118=EDGE_CURVE('',#9039,#9094,#6307,.T.);
#12119=EDGE_CURVE('',#9095,#9096,#5424,.T.);
#12120=EDGE_CURVE('',#9096,#9097,#6308,.T.);
#12121=EDGE_CURVE('',#9097,#9098,#4646,.T.);
#12122=EDGE_CURVE('',#9098,#9099,#6309,.T.);
#12123=EDGE_CURVE('',#9099,#9095,#241,.F.);
#12124=EDGE_CURVE('',#9091,#9100,#4647,.T.);
#12125=EDGE_CURVE('',#9100,#9097,#4648,.T.);
#12126=EDGE_CURVE('',#9097,#9092,#4649,.T.);
#12127=EDGE_CURVE('',#9100,#9098,#4650,.T.);
#12128=EDGE_CURVE('',#9100,#8905,#6310,.T.);
#12129=EDGE_CURVE('',#8904,#9098,#6311,.T.);
#12130=EDGE_CURVE('',#9093,#9096,#4651,.T.);
#12131=EDGE_CURVE('',#9082,#9101,#5425,.F.);
#12132=EDGE_CURVE('',#9101,#9094,#5426,.T.);
#12133=EDGE_CURVE('',#9040,#9101,#6312,.T.);
#12134=EDGE_CURVE('',#9081,#9102,#5427,.T.);
#12135=EDGE_CURVE('',#9089,#9102,#4652,.T.);
#12136=EDGE_CURVE('',#9103,#9102,#6313,.T.);
#12137=EDGE_CURVE('',#9103,#9088,#4653,.T.);
#12138=EDGE_CURVE('',#9087,#9104,#4654,.T.);
#12139=EDGE_CURVE('',#9104,#9103,#5428,.T.);
#12140=EDGE_CURVE('',#9061,#9090,#5429,.T.);
#12141=EDGE_CURVE('',#9085,#9064,#4655,.T.);
#12142=EDGE_CURVE('',#9065,#9084,#4656,.T.);
#12143=EDGE_CURVE('',#9083,#9066,#4657,.T.);
#12144=EDGE_CURVE('',#9076,#9105,#5430,.F.);
#12145=EDGE_CURVE('',#9105,#9086,#5431,.T.);
#12146=EDGE_CURVE('',#9046,#9105,#6314,.T.);
#12147=EDGE_CURVE('',#9106,#9107,#6315,.T.);
#12148=EDGE_CURVE('',#9108,#9107,#4658,.T.);
#12149=EDGE_CURVE('',#9109,#9108,#6316,.T.);
#12150=EDGE_CURVE('',#9106,#9109,#4659,.T.);
#12151=EDGE_CURVE('',#9110,#9106,#5432,.T.);
#12152=EDGE_CURVE('',#9109,#9111,#4660,.T.);
#12153=EDGE_CURVE('',#9111,#9110,#4661,.T.);
#12154=EDGE_CURVE('',#9108,#9112,#5433,.T.);
#12155=EDGE_CURVE('',#9113,#9112,#242,.T.);
#12156=EDGE_CURVE('',#9113,#9114,#6317,.T.);
#12157=EDGE_CURVE('',#9114,#9109,#4662,.T.);
#12158=EDGE_CURVE('',#9114,#9111,#4663,.T.);
#12159=EDGE_CURVE('',#8900,#9111,#6318,.T.);
#12160=EDGE_CURVE('',#8899,#9110,#6319,.T.);
#12161=EDGE_CURVE('',#9114,#8901,#6320,.T.);
#12162=EDGE_CURVE('',#9115,#9113,#6321,.T.);
#12163=EDGE_CURVE('',#9116,#9115,#6322,.T.);
#12164=EDGE_CURVE('',#9117,#9116,#5434,.T.);
#12165=EDGE_CURVE('',#8871,#9117,#6323,.T.);
#12166=EDGE_CURVE('',#9118,#8870,#4664,.F.);
#12167=EDGE_CURVE('',#9118,#9119,#6324,.T.);
#12168=EDGE_CURVE('',#8902,#9119,#4665,.F.);
#12169=EDGE_CURVE('',#9120,#9095,#5435,.T.);
#12170=EDGE_CURVE('',#9120,#9121,#5436,.T.);
#12171=EDGE_CURVE('',#9112,#9121,#5437,.T.);
#12172=EDGE_CURVE('',#9075,#9107,#5438,.T.);
#12173=EDGE_CURVE('',#9099,#9113,#6325,.T.);
#12174=EDGE_CURVE('',#9122,#8903,#4666,.F.);
#12175=EDGE_CURVE('',#9123,#9122,#6326,.T.);
#12176=EDGE_CURVE('',#8869,#9123,#4667,.F.);
#12177=EDGE_CURVE('',#9124,#8868,#6327,.T.);
#12178=EDGE_CURVE('',#9125,#9124,#5439,.T.);
#12179=EDGE_CURVE('',#9126,#9125,#6328,.T.);
#12180=EDGE_CURVE('',#9126,#9099,#6329,.T.);
#12181=EDGE_CURVE('',#9115,#9126,#6330,.T.);
#12182=EDGE_CURVE('',#9123,#9118,#6331,.T.);
#12183=EDGE_CURVE('',#9119,#9122,#6332,.T.);
#12184=EDGE_CURVE('',#9117,#9032,#5440,.T.);
#12185=EDGE_CURVE('',#9033,#9124,#5441,.T.);
#12186=EDGE_CURVE('',#9116,#9125,#4668,.T.);
#12187=EDGE_CURVE('',#8891,#9104,#6333,.T.);
#17440=ORIENTED_EDGE('',*,*,#11753,.T.);
#17441=ORIENTED_EDGE('',*,*,#11754,.T.);
#17442=ORIENTED_EDGE('',*,*,#11755,.T.);
#17443=ORIENTED_EDGE('',*,*,#11756,.T.);
#17444=ORIENTED_EDGE('',*,*,#11754,.F.);
#17445=ORIENTED_EDGE('',*,*,#11757,.F.);
#17446=ORIENTED_EDGE('',*,*,#11758,.F.);
#17447=ORIENTED_EDGE('',*,*,#11759,.T.);
#17448=ORIENTED_EDGE('',*,*,#11755,.F.);
#17449=ORIENTED_EDGE('',*,*,#11756,.F.);
#17450=ORIENTED_EDGE('',*,*,#11759,.F.);
#17451=ORIENTED_EDGE('',*,*,#11760,.T.);
#17452=ORIENTED_EDGE('',*,*,#11761,.F.);
#17453=ORIENTED_EDGE('',*,*,#11762,.F.);
#17454=ORIENTED_EDGE('',*,*,#11763,.F.);
#17455=ORIENTED_EDGE('',*,*,#11764,.T.);
#17456=ORIENTED_EDGE('',*,*,#11765,.F.);
#17457=ORIENTED_EDGE('',*,*,#11766,.T.);
#17458=ORIENTED_EDGE('',*,*,#11767,.F.);
#17459=ORIENTED_EDGE('',*,*,#11768,.F.);
#17460=ORIENTED_EDGE('',*,*,#11769,.F.);
#17461=ORIENTED_EDGE('',*,*,#11770,.F.);
#17462=ORIENTED_EDGE('',*,*,#11771,.T.);
#17463=ORIENTED_EDGE('',*,*,#11772,.F.);
#17464=ORIENTED_EDGE('',*,*,#11773,.T.);
#17465=ORIENTED_EDGE('',*,*,#11774,.F.);
#17466=ORIENTED_EDGE('',*,*,#11775,.F.);
#17467=ORIENTED_EDGE('',*,*,#11776,.F.);
#17468=ORIENTED_EDGE('',*,*,#11777,.T.);
#17469=ORIENTED_EDGE('',*,*,#11778,.F.);
#17470=ORIENTED_EDGE('',*,*,#11779,.T.);
#17471=ORIENTED_EDGE('',*,*,#11780,.F.);
#17472=ORIENTED_EDGE('',*,*,#11781,.F.);
#17473=ORIENTED_EDGE('',*,*,#11782,.F.);
#17474=ORIENTED_EDGE('',*,*,#11783,.T.);
#17475=ORIENTED_EDGE('',*,*,#11784,.F.);
#17476=ORIENTED_EDGE('',*,*,#11753,.F.);
#17477=ORIENTED_EDGE('',*,*,#11757,.T.);
#17478=ORIENTED_EDGE('',*,*,#11758,.T.);
#17479=ORIENTED_EDGE('',*,*,#11785,.T.);
#17480=ORIENTED_EDGE('',*,*,#11786,.T.);
#17481=ORIENTED_EDGE('',*,*,#11785,.F.);
#17482=ORIENTED_EDGE('',*,*,#11787,.T.);
#17483=ORIENTED_EDGE('',*,*,#11788,.T.);
#17484=ORIENTED_EDGE('',*,*,#11789,.T.);
#17485=ORIENTED_EDGE('',*,*,#11790,.F.);
#17486=ORIENTED_EDGE('',*,*,#11791,.T.);
#17487=ORIENTED_EDGE('',*,*,#11792,.T.);
#17488=ORIENTED_EDGE('',*,*,#11793,.T.);
#17489=ORIENTED_EDGE('',*,*,#11794,.F.);
#17490=ORIENTED_EDGE('',*,*,#11795,.T.);
#17491=ORIENTED_EDGE('',*,*,#11796,.T.);
#17492=ORIENTED_EDGE('',*,*,#11797,.F.);
#17493=ORIENTED_EDGE('',*,*,#11798,.T.);
#17494=ORIENTED_EDGE('',*,*,#11799,.F.);
#17495=ORIENTED_EDGE('',*,*,#11800,.T.);
#17496=ORIENTED_EDGE('',*,*,#11801,.F.);
#17497=ORIENTED_EDGE('',*,*,#11802,.T.);
#17498=ORIENTED_EDGE('',*,*,#11803,.T.);
#17499=ORIENTED_EDGE('',*,*,#11804,.F.);
#17500=ORIENTED_EDGE('',*,*,#11786,.F.);
#17501=ORIENTED_EDGE('',*,*,#11805,.T.);
#17502=ORIENTED_EDGE('',*,*,#11806,.T.);
#17503=ORIENTED_EDGE('',*,*,#11807,.T.);
#17504=ORIENTED_EDGE('',*,*,#11784,.T.);
#17505=ORIENTED_EDGE('',*,*,#11806,.F.);
#17506=ORIENTED_EDGE('',*,*,#11808,.T.);
#17507=ORIENTED_EDGE('',*,*,#11809,.F.);
#17508=ORIENTED_EDGE('',*,*,#11810,.F.);
#17509=ORIENTED_EDGE('',*,*,#11811,.T.);
#17510=ORIENTED_EDGE('',*,*,#11809,.T.);
#17511=ORIENTED_EDGE('',*,*,#11812,.T.);
#17512=ORIENTED_EDGE('',*,*,#11804,.T.);
#17513=ORIENTED_EDGE('',*,*,#11813,.T.);
#17514=ORIENTED_EDGE('',*,*,#11814,.T.);
#17515=ORIENTED_EDGE('',*,*,#11815,.T.);
#17516=ORIENTED_EDGE('',*,*,#11778,.T.);
#17517=ORIENTED_EDGE('',*,*,#11814,.F.);
#17518=ORIENTED_EDGE('',*,*,#11816,.T.);
#17519=ORIENTED_EDGE('',*,*,#11817,.F.);
#17520=ORIENTED_EDGE('',*,*,#11818,.F.);
#17521=ORIENTED_EDGE('',*,*,#11819,.T.);
#17522=ORIENTED_EDGE('',*,*,#11817,.T.);
#17523=ORIENTED_EDGE('',*,*,#11820,.T.);
#17524=ORIENTED_EDGE('',*,*,#11790,.T.);
#17525=ORIENTED_EDGE('',*,*,#11821,.T.);
#17526=ORIENTED_EDGE('',*,*,#11822,.T.);
#17527=ORIENTED_EDGE('',*,*,#11823,.T.);
#17528=ORIENTED_EDGE('',*,*,#11772,.T.);
#17529=ORIENTED_EDGE('',*,*,#11822,.F.);
#17530=ORIENTED_EDGE('',*,*,#11824,.T.);
#17531=ORIENTED_EDGE('',*,*,#11825,.F.);
#17532=ORIENTED_EDGE('',*,*,#11826,.F.);
#17533=ORIENTED_EDGE('',*,*,#11827,.T.);
#17534=ORIENTED_EDGE('',*,*,#11825,.T.);
#17535=ORIENTED_EDGE('',*,*,#11828,.T.);
#17536=ORIENTED_EDGE('',*,*,#11794,.T.);
#17537=ORIENTED_EDGE('',*,*,#11829,.T.);
#17538=ORIENTED_EDGE('',*,*,#11830,.T.);
#17539=ORIENTED_EDGE('',*,*,#11831,.T.);
#17540=ORIENTED_EDGE('',*,*,#11832,.T.);
#17541=ORIENTED_EDGE('',*,*,#11831,.F.);
#17542=ORIENTED_EDGE('',*,*,#11833,.T.);
#17543=ORIENTED_EDGE('',*,*,#11834,.T.);
#17544=ORIENTED_EDGE('',*,*,#11835,.T.);
#17545=ORIENTED_EDGE('',*,*,#11836,.T.);
#17546=ORIENTED_EDGE('',*,*,#11837,.T.);
#17547=ORIENTED_EDGE('',*,*,#11838,.T.);
#17548=ORIENTED_EDGE('',*,*,#11837,.F.);
#17549=ORIENTED_EDGE('',*,*,#11839,.T.);
#17550=ORIENTED_EDGE('',*,*,#11840,.T.);
#17551=ORIENTED_EDGE('',*,*,#11835,.F.);
#17552=ORIENTED_EDGE('',*,*,#11841,.T.);
#17553=ORIENTED_EDGE('',*,*,#11829,.F.);
#17554=ORIENTED_EDGE('',*,*,#11834,.F.);
#17555=ORIENTED_EDGE('',*,*,#11842,.T.);
#17556=ORIENTED_EDGE('',*,*,#11843,.T.);
#17557=ORIENTED_EDGE('',*,*,#11844,.T.);
#17558=ORIENTED_EDGE('',*,*,#11833,.F.);
#17559=ORIENTED_EDGE('',*,*,#11845,.T.);
#17560=ORIENTED_EDGE('',*,*,#11846,.F.);
#17561=ORIENTED_EDGE('',*,*,#11847,.T.);
#17562=ORIENTED_EDGE('',*,*,#11830,.F.);
#17563=ORIENTED_EDGE('',*,*,#11848,.F.);
#17564=ORIENTED_EDGE('',*,*,#11849,.F.);
#17565=ORIENTED_EDGE('',*,*,#11845,.F.);
#17566=ORIENTED_EDGE('',*,*,#11841,.F.);
#17567=ORIENTED_EDGE('',*,*,#11850,.T.);
#17568=ORIENTED_EDGE('',*,*,#11851,.T.);
#17569=ORIENTED_EDGE('',*,*,#11848,.T.);
#17570=ORIENTED_EDGE('',*,*,#11838,.F.);
#17571=ORIENTED_EDGE('',*,*,#11852,.F.);
#17572=ORIENTED_EDGE('',*,*,#11853,.F.);
#17573=ORIENTED_EDGE('',*,*,#11854,.T.);
#17574=ORIENTED_EDGE('',*,*,#11855,.F.);
#17575=ORIENTED_EDGE('',*,*,#11850,.F.);
#17576=ORIENTED_EDGE('',*,*,#11856,.F.);
#17577=ORIENTED_EDGE('',*,*,#11857,.T.);
#17578=ORIENTED_EDGE('',*,*,#11858,.T.);
#17579=ORIENTED_EDGE('',*,*,#11855,.T.);
#17580=ORIENTED_EDGE('',*,*,#11859,.F.);
#17581=ORIENTED_EDGE('',*,*,#11858,.F.);
#17582=ORIENTED_EDGE('',*,*,#11860,.T.);
#17583=ORIENTED_EDGE('',*,*,#11851,.F.);
#17584=ORIENTED_EDGE('',*,*,#11832,.F.);
#17585=ORIENTED_EDGE('',*,*,#11844,.F.);
#17586=ORIENTED_EDGE('',*,*,#11861,.F.);
#17587=ORIENTED_EDGE('',*,*,#11836,.F.);
#17588=ORIENTED_EDGE('',*,*,#11860,.F.);
#17589=ORIENTED_EDGE('',*,*,#11862,.T.);
#17590=ORIENTED_EDGE('',*,*,#11863,.F.);
#17591=ORIENTED_EDGE('',*,*,#11849,.T.);
#17592=ORIENTED_EDGE('',*,*,#11864,.F.);
#17593=ORIENTED_EDGE('',*,*,#11865,.T.);
#17594=ORIENTED_EDGE('',*,*,#11866,.T.);
#17595=ORIENTED_EDGE('',*,*,#11867,.F.);
#17596=ORIENTED_EDGE('',*,*,#11868,.T.);
#17597=ORIENTED_EDGE('',*,*,#11869,.F.);
#17598=ORIENTED_EDGE('',*,*,#11870,.F.);
#17599=ORIENTED_EDGE('',*,*,#11871,.F.);
#17600=ORIENTED_EDGE('',*,*,#11872,.F.);
#17601=ORIENTED_EDGE('',*,*,#11873,.F.);
#17602=ORIENTED_EDGE('',*,*,#11874,.T.);
#17603=ORIENTED_EDGE('',*,*,#11875,.F.);
#17604=ORIENTED_EDGE('',*,*,#11876,.F.);
#17605=ORIENTED_EDGE('',*,*,#11877,.F.);
#17606=ORIENTED_EDGE('',*,*,#11878,.F.);
#17607=ORIENTED_EDGE('',*,*,#11879,.F.);
#17608=ORIENTED_EDGE('',*,*,#11862,.F.);
#17609=ORIENTED_EDGE('',*,*,#11857,.F.);
#17610=ORIENTED_EDGE('',*,*,#11880,.T.);
#17611=ORIENTED_EDGE('',*,*,#11865,.F.);
#17612=ORIENTED_EDGE('',*,*,#11881,.F.);
#17613=ORIENTED_EDGE('',*,*,#11882,.T.);
#17614=ORIENTED_EDGE('',*,*,#11883,.T.);
#17615=ORIENTED_EDGE('',*,*,#11884,.T.);
#17616=ORIENTED_EDGE('',*,*,#11875,.T.);
#17617=ORIENTED_EDGE('',*,*,#11885,.T.);
#17618=ORIENTED_EDGE('',*,*,#11886,.T.);
#17619=ORIENTED_EDGE('',*,*,#11887,.T.);
#17620=ORIENTED_EDGE('',*,*,#11884,.F.);
#17621=ORIENTED_EDGE('',*,*,#11888,.T.);
#17622=ORIENTED_EDGE('',*,*,#11889,.T.);
#17623=ORIENTED_EDGE('',*,*,#11890,.T.);
#17624=ORIENTED_EDGE('',*,*,#11888,.F.);
#17625=ORIENTED_EDGE('',*,*,#11891,.T.);
#17626=ORIENTED_EDGE('',*,*,#11886,.F.);
#17627=ORIENTED_EDGE('',*,*,#11892,.T.);
#17628=ORIENTED_EDGE('',*,*,#11887,.F.);
#17629=ORIENTED_EDGE('',*,*,#11893,.T.);
#17630=ORIENTED_EDGE('',*,*,#11894,.F.);
#17631=ORIENTED_EDGE('',*,*,#11876,.T.);
#17632=ORIENTED_EDGE('',*,*,#11891,.F.);
#17633=ORIENTED_EDGE('',*,*,#11895,.F.);
#17634=ORIENTED_EDGE('',*,*,#11896,.F.);
#17635=ORIENTED_EDGE('',*,*,#11893,.F.);
#17636=ORIENTED_EDGE('',*,*,#11890,.F.);
#17637=ORIENTED_EDGE('',*,*,#11897,.T.);
#17638=ORIENTED_EDGE('',*,*,#11898,.T.);
#17639=ORIENTED_EDGE('',*,*,#11895,.T.);
#17640=ORIENTED_EDGE('',*,*,#11899,.T.);
#17641=ORIENTED_EDGE('',*,*,#11900,.T.);
#17642=ORIENTED_EDGE('',*,*,#11885,.F.);
#17643=ORIENTED_EDGE('',*,*,#11874,.F.);
#17644=ORIENTED_EDGE('',*,*,#11900,.F.);
#17645=ORIENTED_EDGE('',*,*,#11901,.F.);
#17646=ORIENTED_EDGE('',*,*,#11902,.F.);
#17647=ORIENTED_EDGE('',*,*,#11903,.F.);
#17648=ORIENTED_EDGE('',*,*,#11904,.F.);
#17649=ORIENTED_EDGE('',*,*,#11882,.F.);
#17650=ORIENTED_EDGE('',*,*,#11905,.T.);
#17651=ORIENTED_EDGE('',*,*,#11906,.T.);
#17652=ORIENTED_EDGE('',*,*,#11907,.T.);
#17653=ORIENTED_EDGE('',*,*,#11908,.T.);
#17654=ORIENTED_EDGE('',*,*,#11909,.T.);
#17655=ORIENTED_EDGE('',*,*,#11910,.T.);
#17656=ORIENTED_EDGE('',*,*,#11872,.T.);
#17657=ORIENTED_EDGE('',*,*,#11911,.T.);
#17658=ORIENTED_EDGE('',*,*,#11908,.F.);
#17659=ORIENTED_EDGE('',*,*,#11912,.T.);
#17660=ORIENTED_EDGE('',*,*,#11913,.T.);
#17661=ORIENTED_EDGE('',*,*,#11914,.T.);
#17662=ORIENTED_EDGE('',*,*,#11910,.F.);
#17663=ORIENTED_EDGE('',*,*,#11915,.T.);
#17664=ORIENTED_EDGE('',*,*,#11916,.T.);
#17665=ORIENTED_EDGE('',*,*,#11917,.T.);
#17666=ORIENTED_EDGE('',*,*,#11915,.F.);
#17667=ORIENTED_EDGE('',*,*,#11918,.T.);
#17668=ORIENTED_EDGE('',*,*,#11913,.F.);
#17669=ORIENTED_EDGE('',*,*,#11919,.T.);
#17670=ORIENTED_EDGE('',*,*,#11911,.F.);
#17671=ORIENTED_EDGE('',*,*,#11920,.T.);
#17672=ORIENTED_EDGE('',*,*,#11905,.F.);
#17673=ORIENTED_EDGE('',*,*,#11921,.T.);
#17674=ORIENTED_EDGE('',*,*,#11912,.F.);
#17675=ORIENTED_EDGE('',*,*,#11871,.T.);
#17676=ORIENTED_EDGE('',*,*,#11922,.F.);
#17677=ORIENTED_EDGE('',*,*,#11923,.T.);
#17678=ORIENTED_EDGE('',*,*,#11924,.T.);
#17679=ORIENTED_EDGE('',*,*,#11914,.F.);
#17680=ORIENTED_EDGE('',*,*,#11925,.T.);
#17681=ORIENTED_EDGE('',*,*,#11901,.T.);
#17682=ORIENTED_EDGE('',*,*,#11899,.F.);
#17683=ORIENTED_EDGE('',*,*,#11873,.T.);
#17684=ORIENTED_EDGE('',*,*,#11918,.F.);
#17685=ORIENTED_EDGE('',*,*,#11926,.F.);
#17686=ORIENTED_EDGE('',*,*,#11927,.F.);
#17687=ORIENTED_EDGE('',*,*,#11928,.T.);
#17688=ORIENTED_EDGE('',*,*,#11902,.T.);
#17689=ORIENTED_EDGE('',*,*,#11925,.F.);
#17690=ORIENTED_EDGE('',*,*,#11917,.F.);
#17691=ORIENTED_EDGE('',*,*,#11929,.T.);
#17692=ORIENTED_EDGE('',*,*,#11930,.T.);
#17693=ORIENTED_EDGE('',*,*,#11926,.T.);
#17694=ORIENTED_EDGE('',*,*,#11931,.T.);
#17695=ORIENTED_EDGE('',*,*,#11932,.T.);
#17696=ORIENTED_EDGE('',*,*,#11866,.F.);
#17697=ORIENTED_EDGE('',*,*,#11880,.F.);
#17698=ORIENTED_EDGE('',*,*,#11856,.T.);
#17699=ORIENTED_EDGE('',*,*,#11931,.F.);
#17700=ORIENTED_EDGE('',*,*,#11859,.T.);
#17701=ORIENTED_EDGE('',*,*,#11854,.F.);
#17702=ORIENTED_EDGE('',*,*,#11933,.F.);
#17703=ORIENTED_EDGE('',*,*,#11934,.F.);
#17704=ORIENTED_EDGE('',*,*,#11935,.F.);
#17705=ORIENTED_EDGE('',*,*,#11846,.T.);
#17706=ORIENTED_EDGE('',*,*,#11863,.T.);
#17707=ORIENTED_EDGE('',*,*,#11936,.T.);
#17708=ORIENTED_EDGE('',*,*,#11843,.F.);
#17709=ORIENTED_EDGE('',*,*,#11937,.T.);
#17710=ORIENTED_EDGE('',*,*,#11938,.T.);
#17711=ORIENTED_EDGE('',*,*,#11937,.F.);
#17712=ORIENTED_EDGE('',*,*,#11939,.T.);
#17713=ORIENTED_EDGE('',*,*,#11940,.T.);
#17714=ORIENTED_EDGE('',*,*,#11941,.T.);
#17715=ORIENTED_EDGE('',*,*,#11847,.F.);
#17716=ORIENTED_EDGE('',*,*,#11942,.F.);
#17717=ORIENTED_EDGE('',*,*,#11943,.T.);
#17718=ORIENTED_EDGE('',*,*,#11944,.F.);
#17719=ORIENTED_EDGE('',*,*,#11939,.F.);
#17720=ORIENTED_EDGE('',*,*,#11842,.F.);
#17721=ORIENTED_EDGE('',*,*,#11936,.F.);
#17722=ORIENTED_EDGE('',*,*,#11879,.T.);
#17723=ORIENTED_EDGE('',*,*,#11945,.T.);
#17724=ORIENTED_EDGE('',*,*,#11946,.T.);
#17725=ORIENTED_EDGE('',*,*,#11942,.T.);
#17726=ORIENTED_EDGE('',*,*,#11947,.T.);
#17727=ORIENTED_EDGE('',*,*,#11898,.F.);
#17728=ORIENTED_EDGE('',*,*,#11948,.T.);
#17729=ORIENTED_EDGE('',*,*,#11949,.T.);
#17730=ORIENTED_EDGE('',*,*,#11896,.T.);
#17731=ORIENTED_EDGE('',*,*,#11947,.F.);
#17732=ORIENTED_EDGE('',*,*,#11950,.T.);
#17733=ORIENTED_EDGE('',*,*,#11877,.T.);
#17734=ORIENTED_EDGE('',*,*,#11951,.T.);
#17735=ORIENTED_EDGE('',*,*,#11952,.T.);
#17736=ORIENTED_EDGE('',*,*,#11953,.T.);
#17737=ORIENTED_EDGE('',*,*,#11954,.T.);
#17738=ORIENTED_EDGE('',*,*,#11878,.T.);
#17739=ORIENTED_EDGE('',*,*,#11954,.F.);
#17740=ORIENTED_EDGE('',*,*,#11955,.T.);
#17741=ORIENTED_EDGE('',*,*,#11945,.F.);
#17742=ORIENTED_EDGE('',*,*,#11951,.F.);
#17743=ORIENTED_EDGE('',*,*,#11894,.T.);
#17744=ORIENTED_EDGE('',*,*,#11949,.F.);
#17745=ORIENTED_EDGE('',*,*,#11952,.F.);
#17746=ORIENTED_EDGE('',*,*,#11950,.F.);
#17747=ORIENTED_EDGE('',*,*,#11956,.F.);
#17748=ORIENTED_EDGE('',*,*,#11957,.F.);
#17749=ORIENTED_EDGE('',*,*,#11958,.F.);
#17750=ORIENTED_EDGE('',*,*,#11959,.T.);
#17751=ORIENTED_EDGE('',*,*,#11948,.F.);
#17752=ORIENTED_EDGE('',*,*,#11960,.T.);
#17753=ORIENTED_EDGE('',*,*,#11961,.T.);
#17754=ORIENTED_EDGE('',*,*,#11956,.T.);
#17755=ORIENTED_EDGE('',*,*,#11897,.F.);
#17756=ORIENTED_EDGE('',*,*,#11962,.F.);
#17757=ORIENTED_EDGE('',*,*,#11963,.F.);
#17758=ORIENTED_EDGE('',*,*,#11960,.F.);
#17759=ORIENTED_EDGE('',*,*,#11889,.F.);
#17760=ORIENTED_EDGE('',*,*,#11964,.T.);
#17761=ORIENTED_EDGE('',*,*,#11965,.T.);
#17762=ORIENTED_EDGE('',*,*,#11962,.T.);
#17763=ORIENTED_EDGE('',*,*,#11965,.F.);
#17764=ORIENTED_EDGE('',*,*,#11966,.T.);
#17765=ORIENTED_EDGE('',*,*,#11967,.T.);
#17766=ORIENTED_EDGE('',*,*,#11968,.T.);
#17767=ORIENTED_EDGE('',*,*,#11969,.T.);
#17768=ORIENTED_EDGE('',*,*,#11922,.T.);
#17769=ORIENTED_EDGE('',*,*,#11870,.T.);
#17770=ORIENTED_EDGE('',*,*,#11969,.F.);
#17771=ORIENTED_EDGE('',*,*,#11970,.F.);
#17772=ORIENTED_EDGE('',*,*,#11971,.F.);
#17773=ORIENTED_EDGE('',*,*,#11972,.F.);
#17774=ORIENTED_EDGE('',*,*,#11973,.F.);
#17775=ORIENTED_EDGE('',*,*,#11923,.F.);
#17776=ORIENTED_EDGE('',*,*,#11974,.F.);
#17777=ORIENTED_EDGE('',*,*,#11975,.T.);
#17778=ORIENTED_EDGE('',*,*,#11976,.T.);
#17779=ORIENTED_EDGE('',*,*,#11977,.T.);
#17780=ORIENTED_EDGE('',*,*,#11972,.T.);
#17781=ORIENTED_EDGE('',*,*,#11978,.F.);
#17782=ORIENTED_EDGE('',*,*,#11967,.F.);
#17783=ORIENTED_EDGE('',*,*,#11979,.T.);
#17784=ORIENTED_EDGE('',*,*,#11980,.T.);
#17785=ORIENTED_EDGE('',*,*,#11963,.T.);
#17786=ORIENTED_EDGE('',*,*,#11966,.F.);
#17787=ORIENTED_EDGE('',*,*,#11981,.T.);
#17788=ORIENTED_EDGE('',*,*,#11982,.T.);
#17789=ORIENTED_EDGE('',*,*,#11983,.T.);
#17790=ORIENTED_EDGE('',*,*,#11903,.T.);
#17791=ORIENTED_EDGE('',*,*,#11928,.F.);
#17792=ORIENTED_EDGE('',*,*,#11984,.F.);
#17793=ORIENTED_EDGE('',*,*,#11985,.T.);
#17794=ORIENTED_EDGE('',*,*,#11982,.F.);
#17795=ORIENTED_EDGE('',*,*,#11986,.T.);
#17796=ORIENTED_EDGE('',*,*,#11980,.F.);
#17797=ORIENTED_EDGE('',*,*,#11987,.T.);
#17798=ORIENTED_EDGE('',*,*,#11961,.F.);
#17799=ORIENTED_EDGE('',*,*,#11987,.F.);
#17800=ORIENTED_EDGE('',*,*,#11988,.T.);
#17801=ORIENTED_EDGE('',*,*,#11989,.T.);
#17802=ORIENTED_EDGE('',*,*,#11957,.T.);
#17803=ORIENTED_EDGE('',*,*,#11990,.F.);
#17804=ORIENTED_EDGE('',*,*,#11781,.T.);
#17805=ORIENTED_EDGE('',*,*,#11991,.T.);
#17806=ORIENTED_EDGE('',*,*,#11992,.F.);
#17807=ORIENTED_EDGE('',*,*,#11993,.F.);
#17808=ORIENTED_EDGE('',*,*,#11775,.T.);
#17809=ORIENTED_EDGE('',*,*,#11994,.T.);
#17810=ORIENTED_EDGE('',*,*,#11995,.F.);
#17811=ORIENTED_EDGE('',*,*,#11996,.F.);
#17812=ORIENTED_EDGE('',*,*,#11769,.T.);
#17813=ORIENTED_EDGE('',*,*,#11997,.T.);
#17814=ORIENTED_EDGE('',*,*,#11998,.F.);
#17815=ORIENTED_EDGE('',*,*,#11999,.F.);
#17816=ORIENTED_EDGE('',*,*,#12000,.F.);
#17817=ORIENTED_EDGE('',*,*,#11941,.F.);
#17818=ORIENTED_EDGE('',*,*,#12001,.F.);
#17819=ORIENTED_EDGE('',*,*,#11988,.F.);
#17820=ORIENTED_EDGE('',*,*,#11979,.F.);
#17821=ORIENTED_EDGE('',*,*,#11983,.F.);
#17822=ORIENTED_EDGE('',*,*,#11985,.F.);
#17823=ORIENTED_EDGE('',*,*,#12002,.T.);
#17824=ORIENTED_EDGE('',*,*,#12003,.F.);
#17825=ORIENTED_EDGE('',*,*,#12004,.T.);
#17826=ORIENTED_EDGE('',*,*,#11975,.F.);
#17827=ORIENTED_EDGE('',*,*,#12005,.T.);
#17828=ORIENTED_EDGE('',*,*,#12006,.F.);
#17829=ORIENTED_EDGE('',*,*,#12007,.F.);
#17830=ORIENTED_EDGE('',*,*,#12008,.F.);
#17831=ORIENTED_EDGE('',*,*,#11997,.F.);
#17832=ORIENTED_EDGE('',*,*,#11768,.T.);
#17833=ORIENTED_EDGE('',*,*,#12009,.F.);
#17834=ORIENTED_EDGE('',*,*,#12010,.F.);
#17835=ORIENTED_EDGE('',*,*,#12011,.F.);
#17836=ORIENTED_EDGE('',*,*,#11762,.T.);
#17837=ORIENTED_EDGE('',*,*,#12012,.T.);
#17838=ORIENTED_EDGE('',*,*,#12013,.F.);
#17839=ORIENTED_EDGE('',*,*,#12014,.T.);
#17840=ORIENTED_EDGE('',*,*,#11782,.T.);
#17841=ORIENTED_EDGE('',*,*,#11990,.T.);
#17842=ORIENTED_EDGE('',*,*,#12015,.T.);
#17843=ORIENTED_EDGE('',*,*,#12013,.T.);
#17844=ORIENTED_EDGE('',*,*,#12016,.T.);
#17845=ORIENTED_EDGE('',*,*,#12017,.T.);
#17846=ORIENTED_EDGE('',*,*,#12018,.T.);
#17847=ORIENTED_EDGE('',*,*,#12019,.T.);
#17848=ORIENTED_EDGE('',*,*,#12015,.F.);
#17849=ORIENTED_EDGE('',*,*,#12018,.F.);
#17850=ORIENTED_EDGE('',*,*,#12020,.T.);
#17851=ORIENTED_EDGE('',*,*,#12021,.T.);
#17852=ORIENTED_EDGE('',*,*,#12022,.T.);
#17853=ORIENTED_EDGE('',*,*,#12023,.T.);
#17854=ORIENTED_EDGE('',*,*,#11770,.T.);
#17855=ORIENTED_EDGE('',*,*,#11996,.T.);
#17856=ORIENTED_EDGE('',*,*,#12024,.T.);
#17857=ORIENTED_EDGE('',*,*,#11995,.T.);
#17858=ORIENTED_EDGE('',*,*,#12025,.T.);
#17859=ORIENTED_EDGE('',*,*,#12026,.T.);
#17860=ORIENTED_EDGE('',*,*,#12027,.T.);
#17861=ORIENTED_EDGE('',*,*,#12028,.T.);
#17862=ORIENTED_EDGE('',*,*,#12024,.F.);
#17863=ORIENTED_EDGE('',*,*,#12027,.F.);
#17864=ORIENTED_EDGE('',*,*,#12029,.T.);
#17865=ORIENTED_EDGE('',*,*,#12030,.T.);
#17866=ORIENTED_EDGE('',*,*,#12031,.T.);
#17867=ORIENTED_EDGE('',*,*,#11840,.F.);
#17868=ORIENTED_EDGE('',*,*,#11999,.T.);
#17869=ORIENTED_EDGE('',*,*,#12032,.T.);
#17870=ORIENTED_EDGE('',*,*,#11852,.T.);
#17871=ORIENTED_EDGE('',*,*,#12006,.T.);
#17872=ORIENTED_EDGE('',*,*,#12033,.T.);
#17873=ORIENTED_EDGE('',*,*,#12034,.T.);
#17874=ORIENTED_EDGE('',*,*,#12035,.T.);
#17875=ORIENTED_EDGE('',*,*,#12036,.T.);
#17876=ORIENTED_EDGE('',*,*,#12033,.F.);
#17877=ORIENTED_EDGE('',*,*,#12037,.T.);
#17878=ORIENTED_EDGE('',*,*,#12038,.T.);
#17879=ORIENTED_EDGE('',*,*,#12007,.T.);
#17880=ORIENTED_EDGE('',*,*,#12036,.F.);
#17881=ORIENTED_EDGE('',*,*,#12039,.T.);
#17882=ORIENTED_EDGE('',*,*,#12040,.T.);
#17883=ORIENTED_EDGE('',*,*,#11998,.T.);
#17884=ORIENTED_EDGE('',*,*,#12008,.T.);
#17885=ORIENTED_EDGE('',*,*,#12040,.F.);
#17886=ORIENTED_EDGE('',*,*,#12041,.T.);
#17887=ORIENTED_EDGE('',*,*,#11933,.T.);
#17888=ORIENTED_EDGE('',*,*,#11853,.T.);
#17889=ORIENTED_EDGE('',*,*,#12032,.F.);
#17890=ORIENTED_EDGE('',*,*,#11839,.F.);
#17891=ORIENTED_EDGE('',*,*,#11861,.T.);
#17892=ORIENTED_EDGE('',*,*,#11938,.F.);
#17893=ORIENTED_EDGE('',*,*,#12000,.T.);
#17894=ORIENTED_EDGE('',*,*,#12001,.T.);
#17895=ORIENTED_EDGE('',*,*,#11940,.F.);
#17896=ORIENTED_EDGE('',*,*,#11944,.T.);
#17897=ORIENTED_EDGE('',*,*,#12042,.T.);
#17898=ORIENTED_EDGE('',*,*,#11958,.T.);
#17899=ORIENTED_EDGE('',*,*,#11989,.F.);
#17900=ORIENTED_EDGE('',*,*,#11955,.F.);
#17901=ORIENTED_EDGE('',*,*,#11953,.F.);
#17902=ORIENTED_EDGE('',*,*,#11959,.F.);
#17903=ORIENTED_EDGE('',*,*,#12042,.F.);
#17904=ORIENTED_EDGE('',*,*,#11943,.F.);
#17905=ORIENTED_EDGE('',*,*,#11946,.F.);
#17906=ORIENTED_EDGE('',*,*,#12037,.F.);
#17907=ORIENTED_EDGE('',*,*,#12005,.F.);
#17908=ORIENTED_EDGE('',*,*,#11974,.T.);
#17909=ORIENTED_EDGE('',*,*,#12043,.T.);
#17910=ORIENTED_EDGE('',*,*,#12038,.F.);
#17911=ORIENTED_EDGE('',*,*,#12044,.T.);
#17912=ORIENTED_EDGE('',*,*,#12045,.T.);
#17913=ORIENTED_EDGE('',*,*,#12046,.T.);
#17914=ORIENTED_EDGE('',*,*,#12047,.T.);
#17915=ORIENTED_EDGE('',*,*,#12045,.F.);
#17916=ORIENTED_EDGE('',*,*,#12048,.T.);
#17917=ORIENTED_EDGE('',*,*,#12048,.F.);
#17918=ORIENTED_EDGE('',*,*,#12049,.T.);
#17919=ORIENTED_EDGE('',*,*,#11970,.T.);
#17920=ORIENTED_EDGE('',*,*,#11968,.F.);
#17921=ORIENTED_EDGE('',*,*,#11869,.T.);
#17922=ORIENTED_EDGE('',*,*,#12044,.F.);
#17923=ORIENTED_EDGE('',*,*,#12043,.F.);
#17924=ORIENTED_EDGE('',*,*,#11978,.T.);
#17925=ORIENTED_EDGE('',*,*,#11971,.T.);
#17926=ORIENTED_EDGE('',*,*,#12049,.F.);
#17927=ORIENTED_EDGE('',*,*,#11907,.F.);
#17928=ORIENTED_EDGE('',*,*,#12050,.T.);
#17929=ORIENTED_EDGE('',*,*,#11916,.F.);
#17930=ORIENTED_EDGE('',*,*,#12051,.T.);
#17931=ORIENTED_EDGE('',*,*,#12050,.F.);
#17932=ORIENTED_EDGE('',*,*,#12052,.F.);
#17933=ORIENTED_EDGE('',*,*,#12053,.F.);
#17934=ORIENTED_EDGE('',*,*,#11929,.F.);
#17935=ORIENTED_EDGE('',*,*,#11906,.F.);
#17936=ORIENTED_EDGE('',*,*,#12054,.T.);
#17937=ORIENTED_EDGE('',*,*,#12055,.T.);
#17938=ORIENTED_EDGE('',*,*,#12052,.T.);
#17939=ORIENTED_EDGE('',*,*,#12056,.F.);
#17940=ORIENTED_EDGE('',*,*,#12057,.F.);
#17941=ORIENTED_EDGE('',*,*,#12055,.F.);
#17942=ORIENTED_EDGE('',*,*,#12058,.F.);
#17943=ORIENTED_EDGE('',*,*,#12059,.F.);
#17944=ORIENTED_EDGE('',*,*,#11930,.F.);
#17945=ORIENTED_EDGE('',*,*,#11927,.T.);
#17946=ORIENTED_EDGE('',*,*,#12059,.T.);
#17947=ORIENTED_EDGE('',*,*,#12002,.F.);
#17948=ORIENTED_EDGE('',*,*,#11984,.T.);
#17949=ORIENTED_EDGE('',*,*,#12058,.T.);
#17950=ORIENTED_EDGE('',*,*,#12053,.T.);
#17951=ORIENTED_EDGE('',*,*,#12057,.T.);
#17952=ORIENTED_EDGE('',*,*,#12003,.T.);
#17953=ORIENTED_EDGE('',*,*,#12004,.F.);
#17954=ORIENTED_EDGE('',*,*,#12056,.T.);
#17955=ORIENTED_EDGE('',*,*,#12060,.T.);
#17956=ORIENTED_EDGE('',*,*,#11976,.F.);
#17957=ORIENTED_EDGE('',*,*,#11920,.F.);
#17958=ORIENTED_EDGE('',*,*,#11924,.F.);
#17959=ORIENTED_EDGE('',*,*,#11973,.T.);
#17960=ORIENTED_EDGE('',*,*,#11977,.F.);
#17961=ORIENTED_EDGE('',*,*,#12060,.F.);
#17962=ORIENTED_EDGE('',*,*,#12054,.F.);
#17963=ORIENTED_EDGE('',*,*,#12034,.F.);
#17964=ORIENTED_EDGE('',*,*,#12046,.F.);
#17965=ORIENTED_EDGE('',*,*,#12061,.F.);
#17966=ORIENTED_EDGE('',*,*,#12062,.F.);
#17967=ORIENTED_EDGE('',*,*,#12063,.T.);
#17968=ORIENTED_EDGE('',*,*,#12064,.T.);
#17969=ORIENTED_EDGE('',*,*,#11867,.T.);
#17970=ORIENTED_EDGE('',*,*,#11932,.F.);
#17971=ORIENTED_EDGE('',*,*,#11935,.T.);
#17972=ORIENTED_EDGE('',*,*,#12065,.T.);
#17973=ORIENTED_EDGE('',*,*,#12062,.T.);
#17974=ORIENTED_EDGE('',*,*,#12035,.F.);
#17975=ORIENTED_EDGE('',*,*,#12063,.F.);
#17976=ORIENTED_EDGE('',*,*,#12065,.F.);
#17977=ORIENTED_EDGE('',*,*,#11934,.T.);
#17978=ORIENTED_EDGE('',*,*,#12041,.F.);
#17979=ORIENTED_EDGE('',*,*,#12039,.F.);
#17980=ORIENTED_EDGE('',*,*,#12066,.T.);
#17981=ORIENTED_EDGE('',*,*,#12067,.T.);
#17982=ORIENTED_EDGE('',*,*,#11776,.T.);
#17983=ORIENTED_EDGE('',*,*,#11993,.T.);
#17984=ORIENTED_EDGE('',*,*,#11777,.F.);
#17985=ORIENTED_EDGE('',*,*,#12067,.F.);
#17986=ORIENTED_EDGE('',*,*,#12068,.F.);
#17987=ORIENTED_EDGE('',*,*,#12069,.F.);
#17988=ORIENTED_EDGE('',*,*,#12070,.T.);
#17989=ORIENTED_EDGE('',*,*,#12071,.F.);
#17990=ORIENTED_EDGE('',*,*,#12072,.T.);
#17991=ORIENTED_EDGE('',*,*,#12073,.T.);
#17992=ORIENTED_EDGE('',*,*,#12074,.F.);
#17993=ORIENTED_EDGE('',*,*,#12075,.F.);
#17994=ORIENTED_EDGE('',*,*,#12076,.F.);
#17995=ORIENTED_EDGE('',*,*,#11791,.F.);
#17996=ORIENTED_EDGE('',*,*,#11820,.F.);
#17997=ORIENTED_EDGE('',*,*,#11816,.F.);
#17998=ORIENTED_EDGE('',*,*,#11813,.F.);
#17999=ORIENTED_EDGE('',*,*,#12077,.T.);
#18000=ORIENTED_EDGE('',*,*,#12078,.T.);
#18001=ORIENTED_EDGE('',*,*,#12068,.T.);
#18002=ORIENTED_EDGE('',*,*,#12066,.F.);
#18003=ORIENTED_EDGE('',*,*,#11992,.T.);
#18004=ORIENTED_EDGE('',*,*,#12079,.T.);
#18005=ORIENTED_EDGE('',*,*,#12078,.F.);
#18006=ORIENTED_EDGE('',*,*,#12080,.T.);
#18007=ORIENTED_EDGE('',*,*,#12081,.T.);
#18008=ORIENTED_EDGE('',*,*,#12069,.T.);
#18009=ORIENTED_EDGE('',*,*,#12082,.T.);
#18010=ORIENTED_EDGE('',*,*,#12083,.T.);
#18011=ORIENTED_EDGE('',*,*,#12084,.T.);
#18012=ORIENTED_EDGE('',*,*,#11881,.T.);
#18013=ORIENTED_EDGE('',*,*,#11864,.T.);
#18014=ORIENTED_EDGE('',*,*,#12084,.F.);
#18015=ORIENTED_EDGE('',*,*,#12085,.F.);
#18016=ORIENTED_EDGE('',*,*,#12086,.F.);
#18017=ORIENTED_EDGE('',*,*,#12087,.T.);
#18018=ORIENTED_EDGE('',*,*,#12082,.F.);
#18019=ORIENTED_EDGE('',*,*,#12083,.F.);
#18020=ORIENTED_EDGE('',*,*,#12087,.F.);
#18021=ORIENTED_EDGE('',*,*,#12088,.F.);
#18022=ORIENTED_EDGE('',*,*,#12089,.F.);
#18023=ORIENTED_EDGE('',*,*,#12090,.F.);
#18024=ORIENTED_EDGE('',*,*,#12091,.F.);
#18025=ORIENTED_EDGE('',*,*,#12092,.F.);
#18026=ORIENTED_EDGE('',*,*,#12072,.F.);
#18027=ORIENTED_EDGE('',*,*,#12093,.F.);
#18028=ORIENTED_EDGE('',*,*,#12094,.F.);
#18029=ORIENTED_EDGE('',*,*,#12095,.F.);
#18030=ORIENTED_EDGE('',*,*,#12096,.F.);
#18031=ORIENTED_EDGE('',*,*,#12097,.F.);
#18032=ORIENTED_EDGE('',*,*,#11774,.T.);
#18033=ORIENTED_EDGE('',*,*,#12098,.T.);
#18034=ORIENTED_EDGE('',*,*,#12025,.F.);
#18035=ORIENTED_EDGE('',*,*,#11994,.F.);
#18036=ORIENTED_EDGE('',*,*,#12098,.F.);
#18037=ORIENTED_EDGE('',*,*,#11773,.F.);
#18038=ORIENTED_EDGE('',*,*,#11823,.F.);
#18039=ORIENTED_EDGE('',*,*,#11826,.T.);
#18040=ORIENTED_EDGE('',*,*,#11827,.F.);
#18041=ORIENTED_EDGE('',*,*,#11793,.F.);
#18042=ORIENTED_EDGE('',*,*,#12099,.F.);
#18043=ORIENTED_EDGE('',*,*,#12100,.F.);
#18044=ORIENTED_EDGE('',*,*,#12101,.T.);
#18045=ORIENTED_EDGE('',*,*,#12102,.T.);
#18046=ORIENTED_EDGE('',*,*,#12091,.T.);
#18047=ORIENTED_EDGE('',*,*,#12103,.T.);
#18048=ORIENTED_EDGE('',*,*,#12104,.F.);
#18049=ORIENTED_EDGE('',*,*,#12029,.F.);
#18050=ORIENTED_EDGE('',*,*,#12026,.F.);
#18051=ORIENTED_EDGE('',*,*,#11780,.T.);
#18052=ORIENTED_EDGE('',*,*,#12105,.T.);
#18053=ORIENTED_EDGE('',*,*,#12079,.F.);
#18054=ORIENTED_EDGE('',*,*,#11991,.F.);
#18055=ORIENTED_EDGE('',*,*,#12105,.F.);
#18056=ORIENTED_EDGE('',*,*,#11779,.F.);
#18057=ORIENTED_EDGE('',*,*,#11815,.F.);
#18058=ORIENTED_EDGE('',*,*,#11818,.T.);
#18059=ORIENTED_EDGE('',*,*,#11819,.F.);
#18060=ORIENTED_EDGE('',*,*,#11789,.F.);
#18061=ORIENTED_EDGE('',*,*,#12106,.F.);
#18062=ORIENTED_EDGE('',*,*,#12107,.F.);
#18063=ORIENTED_EDGE('',*,*,#12108,.T.);
#18064=ORIENTED_EDGE('',*,*,#12109,.T.);
#18065=ORIENTED_EDGE('',*,*,#12094,.T.);
#18066=ORIENTED_EDGE('',*,*,#12110,.T.);
#18067=ORIENTED_EDGE('',*,*,#12111,.F.);
#18068=ORIENTED_EDGE('',*,*,#12080,.F.);
#18069=ORIENTED_EDGE('',*,*,#12077,.F.);
#18070=ORIENTED_EDGE('',*,*,#11761,.T.);
#18071=ORIENTED_EDGE('',*,*,#12112,.T.);
#18072=ORIENTED_EDGE('',*,*,#12016,.F.);
#18073=ORIENTED_EDGE('',*,*,#12012,.F.);
#18074=ORIENTED_EDGE('',*,*,#12112,.F.);
#18075=ORIENTED_EDGE('',*,*,#11760,.F.);
#18076=ORIENTED_EDGE('',*,*,#11807,.F.);
#18077=ORIENTED_EDGE('',*,*,#11810,.T.);
#18078=ORIENTED_EDGE('',*,*,#11811,.F.);
#18079=ORIENTED_EDGE('',*,*,#11803,.F.);
#18080=ORIENTED_EDGE('',*,*,#12113,.F.);
#18081=ORIENTED_EDGE('',*,*,#12114,.F.);
#18082=ORIENTED_EDGE('',*,*,#12115,.T.);
#18083=ORIENTED_EDGE('',*,*,#12116,.T.);
#18084=ORIENTED_EDGE('',*,*,#12085,.T.);
#18085=ORIENTED_EDGE('',*,*,#12117,.T.);
#18086=ORIENTED_EDGE('',*,*,#12118,.F.);
#18087=ORIENTED_EDGE('',*,*,#12020,.F.);
#18088=ORIENTED_EDGE('',*,*,#12017,.F.);
#18089=ORIENTED_EDGE('',*,*,#12119,.T.);
#18090=ORIENTED_EDGE('',*,*,#12120,.T.);
#18091=ORIENTED_EDGE('',*,*,#12121,.T.);
#18092=ORIENTED_EDGE('',*,*,#12122,.T.);
#18093=ORIENTED_EDGE('',*,*,#12123,.T.);
#18094=ORIENTED_EDGE('',*,*,#12114,.T.);
#18095=ORIENTED_EDGE('',*,*,#12124,.T.);
#18096=ORIENTED_EDGE('',*,*,#12125,.T.);
#18097=ORIENTED_EDGE('',*,*,#12126,.T.);
#18098=ORIENTED_EDGE('',*,*,#12125,.F.);
#18099=ORIENTED_EDGE('',*,*,#12127,.T.);
#18100=ORIENTED_EDGE('',*,*,#12121,.F.);
#18101=ORIENTED_EDGE('',*,*,#12127,.F.);
#18102=ORIENTED_EDGE('',*,*,#12128,.T.);
#18103=ORIENTED_EDGE('',*,*,#11801,.T.);
#18104=ORIENTED_EDGE('',*,*,#12129,.T.);
#18105=ORIENTED_EDGE('',*,*,#12124,.F.);
#18106=ORIENTED_EDGE('',*,*,#12113,.T.);
#18107=ORIENTED_EDGE('',*,*,#11802,.F.);
#18108=ORIENTED_EDGE('',*,*,#12128,.F.);
#18109=ORIENTED_EDGE('',*,*,#12126,.F.);
#18110=ORIENTED_EDGE('',*,*,#12120,.F.);
#18111=ORIENTED_EDGE('',*,*,#12130,.F.);
#18112=ORIENTED_EDGE('',*,*,#12115,.F.);
#18113=ORIENTED_EDGE('',*,*,#12117,.F.);
#18114=ORIENTED_EDGE('',*,*,#12097,.T.);
#18115=ORIENTED_EDGE('',*,*,#12131,.T.);
#18116=ORIENTED_EDGE('',*,*,#12132,.T.);
#18117=ORIENTED_EDGE('',*,*,#12132,.F.);
#18118=ORIENTED_EDGE('',*,*,#12133,.F.);
#18119=ORIENTED_EDGE('',*,*,#12021,.F.);
#18120=ORIENTED_EDGE('',*,*,#12118,.T.);
#18121=ORIENTED_EDGE('',*,*,#12134,.F.);
#18122=ORIENTED_EDGE('',*,*,#12095,.T.);
#18123=ORIENTED_EDGE('',*,*,#12109,.F.);
#18124=ORIENTED_EDGE('',*,*,#12135,.T.);
#18125=ORIENTED_EDGE('',*,*,#12136,.T.);
#18126=ORIENTED_EDGE('',*,*,#12135,.F.);
#18127=ORIENTED_EDGE('',*,*,#12108,.F.);
#18128=ORIENTED_EDGE('',*,*,#12137,.F.);
#18129=ORIENTED_EDGE('',*,*,#12107,.T.);
#18130=ORIENTED_EDGE('',*,*,#12138,.T.);
#18131=ORIENTED_EDGE('',*,*,#12139,.T.);
#18132=ORIENTED_EDGE('',*,*,#12137,.T.);
#18133=ORIENTED_EDGE('',*,*,#12110,.F.);
#18134=ORIENTED_EDGE('',*,*,#12093,.T.);
#18135=ORIENTED_EDGE('',*,*,#12071,.T.);
#18136=ORIENTED_EDGE('',*,*,#12140,.T.);
#18137=ORIENTED_EDGE('',*,*,#12140,.F.);
#18138=ORIENTED_EDGE('',*,*,#12070,.F.);
#18139=ORIENTED_EDGE('',*,*,#12081,.F.);
#18140=ORIENTED_EDGE('',*,*,#12111,.T.);
#18141=ORIENTED_EDGE('',*,*,#12073,.F.);
#18142=ORIENTED_EDGE('',*,*,#12092,.T.);
#18143=ORIENTED_EDGE('',*,*,#12102,.F.);
#18144=ORIENTED_EDGE('',*,*,#12141,.T.);
#18145=ORIENTED_EDGE('',*,*,#12074,.T.);
#18146=ORIENTED_EDGE('',*,*,#12141,.F.);
#18147=ORIENTED_EDGE('',*,*,#12101,.F.);
#18148=ORIENTED_EDGE('',*,*,#12142,.F.);
#18149=ORIENTED_EDGE('',*,*,#12100,.T.);
#18150=ORIENTED_EDGE('',*,*,#12143,.T.);
#18151=ORIENTED_EDGE('',*,*,#12075,.T.);
#18152=ORIENTED_EDGE('',*,*,#12142,.T.);
#18153=ORIENTED_EDGE('',*,*,#12103,.F.);
#18154=ORIENTED_EDGE('',*,*,#12090,.T.);
#18155=ORIENTED_EDGE('',*,*,#12144,.T.);
#18156=ORIENTED_EDGE('',*,*,#12145,.T.);
#18157=ORIENTED_EDGE('',*,*,#12145,.F.);
#18158=ORIENTED_EDGE('',*,*,#12146,.F.);
#18159=ORIENTED_EDGE('',*,*,#12030,.F.);
#18160=ORIENTED_EDGE('',*,*,#12104,.T.);
#18161=ORIENTED_EDGE('',*,*,#12147,.T.);
#18162=ORIENTED_EDGE('',*,*,#12148,.F.);
#18163=ORIENTED_EDGE('',*,*,#12149,.F.);
#18164=ORIENTED_EDGE('',*,*,#12150,.F.);
#18165=ORIENTED_EDGE('',*,*,#12151,.T.);
#18166=ORIENTED_EDGE('',*,*,#12150,.T.);
#18167=ORIENTED_EDGE('',*,*,#12152,.T.);
#18168=ORIENTED_EDGE('',*,*,#12153,.T.);
#18169=ORIENTED_EDGE('',*,*,#12154,.T.);
#18170=ORIENTED_EDGE('',*,*,#12155,.F.);
#18171=ORIENTED_EDGE('',*,*,#12156,.T.);
#18172=ORIENTED_EDGE('',*,*,#12157,.T.);
#18173=ORIENTED_EDGE('',*,*,#12149,.T.);
#18174=ORIENTED_EDGE('',*,*,#12157,.F.);
#18175=ORIENTED_EDGE('',*,*,#12158,.T.);
#18176=ORIENTED_EDGE('',*,*,#12152,.F.);
#18177=ORIENTED_EDGE('',*,*,#12153,.F.);
#18178=ORIENTED_EDGE('',*,*,#12159,.F.);
#18179=ORIENTED_EDGE('',*,*,#11796,.F.);
#18180=ORIENTED_EDGE('',*,*,#12160,.T.);
#18181=ORIENTED_EDGE('',*,*,#12158,.F.);
#18182=ORIENTED_EDGE('',*,*,#12161,.T.);
#18183=ORIENTED_EDGE('',*,*,#11797,.T.);
#18184=ORIENTED_EDGE('',*,*,#12159,.T.);
#18185=ORIENTED_EDGE('',*,*,#12156,.F.);
#18186=ORIENTED_EDGE('',*,*,#12162,.F.);
#18187=ORIENTED_EDGE('',*,*,#12163,.F.);
#18188=ORIENTED_EDGE('',*,*,#12164,.F.);
#18189=ORIENTED_EDGE('',*,*,#12165,.F.);
#18190=ORIENTED_EDGE('',*,*,#11766,.F.);
#18191=ORIENTED_EDGE('',*,*,#12166,.F.);
#18192=ORIENTED_EDGE('',*,*,#12167,.T.);
#18193=ORIENTED_EDGE('',*,*,#12168,.F.);
#18194=ORIENTED_EDGE('',*,*,#11798,.F.);
#18195=ORIENTED_EDGE('',*,*,#12161,.F.);
#18196=ORIENTED_EDGE('',*,*,#12169,.F.);
#18197=ORIENTED_EDGE('',*,*,#12170,.T.);
#18198=ORIENTED_EDGE('',*,*,#12171,.F.);
#18199=ORIENTED_EDGE('',*,*,#12154,.F.);
#18200=ORIENTED_EDGE('',*,*,#12148,.T.);
#18201=ORIENTED_EDGE('',*,*,#12172,.F.);
#18202=ORIENTED_EDGE('',*,*,#12088,.T.);
#18203=ORIENTED_EDGE('',*,*,#12086,.T.);
#18204=ORIENTED_EDGE('',*,*,#12116,.F.);
#18205=ORIENTED_EDGE('',*,*,#12130,.T.);
#18206=ORIENTED_EDGE('',*,*,#12119,.F.);
#18207=ORIENTED_EDGE('',*,*,#12170,.F.);
#18208=ORIENTED_EDGE('',*,*,#12169,.T.);
#18209=ORIENTED_EDGE('',*,*,#12123,.F.);
#18210=ORIENTED_EDGE('',*,*,#12173,.T.);
#18211=ORIENTED_EDGE('',*,*,#12155,.T.);
#18212=ORIENTED_EDGE('',*,*,#12171,.T.);
#18213=ORIENTED_EDGE('',*,*,#12122,.F.);
#18214=ORIENTED_EDGE('',*,*,#12129,.F.);
#18215=ORIENTED_EDGE('',*,*,#11800,.F.);
#18216=ORIENTED_EDGE('',*,*,#12174,.F.);
#18217=ORIENTED_EDGE('',*,*,#12175,.F.);
#18218=ORIENTED_EDGE('',*,*,#12176,.F.);
#18219=ORIENTED_EDGE('',*,*,#11764,.F.);
#18220=ORIENTED_EDGE('',*,*,#12177,.F.);
#18221=ORIENTED_EDGE('',*,*,#12178,.F.);
#18222=ORIENTED_EDGE('',*,*,#12179,.F.);
#18223=ORIENTED_EDGE('',*,*,#12180,.T.);
#18224=ORIENTED_EDGE('',*,*,#12173,.F.);
#18225=ORIENTED_EDGE('',*,*,#12180,.F.);
#18226=ORIENTED_EDGE('',*,*,#12181,.F.);
#18227=ORIENTED_EDGE('',*,*,#12162,.T.);
#18228=ORIENTED_EDGE('',*,*,#12176,.T.);
#18229=ORIENTED_EDGE('',*,*,#12182,.T.);
#18230=ORIENTED_EDGE('',*,*,#12166,.T.);
#18231=ORIENTED_EDGE('',*,*,#11765,.T.);
#18232=ORIENTED_EDGE('',*,*,#12182,.F.);
#18233=ORIENTED_EDGE('',*,*,#12175,.T.);
#18234=ORIENTED_EDGE('',*,*,#12183,.F.);
#18235=ORIENTED_EDGE('',*,*,#12167,.F.);
#18236=ORIENTED_EDGE('',*,*,#12168,.T.);
#18237=ORIENTED_EDGE('',*,*,#12183,.T.);
#18238=ORIENTED_EDGE('',*,*,#12174,.T.);
#18239=ORIENTED_EDGE('',*,*,#11799,.T.);
#18240=ORIENTED_EDGE('',*,*,#12009,.T.);
#18241=ORIENTED_EDGE('',*,*,#11767,.T.);
#18242=ORIENTED_EDGE('',*,*,#12165,.T.);
#18243=ORIENTED_EDGE('',*,*,#12184,.T.);
#18244=ORIENTED_EDGE('',*,*,#12177,.T.);
#18245=ORIENTED_EDGE('',*,*,#11763,.T.);
#18246=ORIENTED_EDGE('',*,*,#12011,.T.);
#18247=ORIENTED_EDGE('',*,*,#12185,.T.);
#18248=ORIENTED_EDGE('',*,*,#12186,.T.);
#18249=ORIENTED_EDGE('',*,*,#12178,.T.);
#18250=ORIENTED_EDGE('',*,*,#12185,.F.);
#18251=ORIENTED_EDGE('',*,*,#12010,.T.);
#18252=ORIENTED_EDGE('',*,*,#12184,.F.);
#18253=ORIENTED_EDGE('',*,*,#12164,.T.);
#18254=ORIENTED_EDGE('',*,*,#12186,.F.);
#18255=ORIENTED_EDGE('',*,*,#12163,.T.);
#18256=ORIENTED_EDGE('',*,*,#12181,.T.);
#18257=ORIENTED_EDGE('',*,*,#12179,.T.);
#18258=ORIENTED_EDGE('',*,*,#12023,.F.);
#18259=ORIENTED_EDGE('',*,*,#12028,.F.);
#18260=ORIENTED_EDGE('',*,*,#12031,.F.);
#18261=ORIENTED_EDGE('',*,*,#12146,.T.);
#18262=ORIENTED_EDGE('',*,*,#12144,.F.);
#18263=ORIENTED_EDGE('',*,*,#12089,.T.);
#18264=ORIENTED_EDGE('',*,*,#12172,.T.);
#18265=ORIENTED_EDGE('',*,*,#12147,.F.);
#18266=ORIENTED_EDGE('',*,*,#12151,.F.);
#18267=ORIENTED_EDGE('',*,*,#12160,.F.);
#18268=ORIENTED_EDGE('',*,*,#11795,.F.);
#18269=ORIENTED_EDGE('',*,*,#11828,.F.);
#18270=ORIENTED_EDGE('',*,*,#11824,.F.);
#18271=ORIENTED_EDGE('',*,*,#11821,.F.);
#18272=ORIENTED_EDGE('',*,*,#11771,.F.);
#18273=ORIENTED_EDGE('',*,*,#12014,.F.);
#18274=ORIENTED_EDGE('',*,*,#12019,.F.);
#18275=ORIENTED_EDGE('',*,*,#12022,.F.);
#18276=ORIENTED_EDGE('',*,*,#12133,.T.);
#18277=ORIENTED_EDGE('',*,*,#12131,.F.);
#18278=ORIENTED_EDGE('',*,*,#12096,.T.);
#18279=ORIENTED_EDGE('',*,*,#12134,.T.);
#18280=ORIENTED_EDGE('',*,*,#12136,.F.);
#18281=ORIENTED_EDGE('',*,*,#12139,.F.);
#18282=ORIENTED_EDGE('',*,*,#12187,.F.);
#18283=ORIENTED_EDGE('',*,*,#11787,.F.);
#18284=ORIENTED_EDGE('',*,*,#11812,.F.);
#18285=ORIENTED_EDGE('',*,*,#11808,.F.);
#18286=ORIENTED_EDGE('',*,*,#11805,.F.);
#18287=ORIENTED_EDGE('',*,*,#11783,.F.);
#18288=ORIENTED_EDGE('',*,*,#12138,.F.);
#18289=ORIENTED_EDGE('',*,*,#12106,.T.);
#18290=ORIENTED_EDGE('',*,*,#11788,.F.);
#18291=ORIENTED_EDGE('',*,*,#12187,.T.);
#18292=ORIENTED_EDGE('',*,*,#12143,.F.);
#18293=ORIENTED_EDGE('',*,*,#12099,.T.);
#18294=ORIENTED_EDGE('',*,*,#11792,.F.);
#18295=ORIENTED_EDGE('',*,*,#12076,.T.);
#18296=ORIENTED_EDGE('',*,*,#11883,.F.);
#18297=ORIENTED_EDGE('',*,*,#11904,.T.);
#18298=ORIENTED_EDGE('',*,*,#11986,.F.);
#18299=ORIENTED_EDGE('',*,*,#11981,.F.);
#18300=ORIENTED_EDGE('',*,*,#11964,.F.);
#18301=ORIENTED_EDGE('',*,*,#11892,.F.);
#18302=ORIENTED_EDGE('',*,*,#11921,.F.);
#18303=ORIENTED_EDGE('',*,*,#12051,.F.);
#18304=ORIENTED_EDGE('',*,*,#11919,.F.);
#18305=ORIENTED_EDGE('',*,*,#11909,.F.);
#18306=ORIENTED_EDGE('',*,*,#12047,.F.);
#18307=ORIENTED_EDGE('',*,*,#11868,.F.);
#18308=ORIENTED_EDGE('',*,*,#12064,.F.);
#18309=ORIENTED_EDGE('',*,*,#12061,.T.);
#18771=CYLINDRICAL_SURFACE('',#22047,9.);
#18772=CYLINDRICAL_SURFACE('',#22074,0.5);
#18773=CYLINDRICAL_SURFACE('',#22078,0.5);
#18774=CYLINDRICAL_SURFACE('',#22081,0.5);
#18775=CYLINDRICAL_SURFACE('',#22085,0.5);
#18776=CYLINDRICAL_SURFACE('',#22088,0.5);
#18777=CYLINDRICAL_SURFACE('',#22092,0.5);
#18778=CYLINDRICAL_SURFACE('',#22103,0.5);
#18779=CYLINDRICAL_SURFACE('',#22111,0.5);
#18780=CYLINDRICAL_SURFACE('',#22118,0.5);
#18781=CYLINDRICAL_SURFACE('',#22128,21.);
#18782=CYLINDRICAL_SURFACE('',#22139,0.5);
#18783=CYLINDRICAL_SURFACE('',#22180,0.5);
#18784=CYLINDRICAL_SURFACE('',#22182,0.5);
#18785=CYLINDRICAL_SURFACE('',#22184,0.5);
#18786=CYLINDRICAL_SURFACE('',#22196,0.5);
#18787=CYLINDRICAL_SURFACE('',#22198,0.5);
#18788=CYLINDRICAL_SURFACE('',#22204,0.5);
#18789=CYLINDRICAL_SURFACE('',#22211,0.5);
#18790=CYLINDRICAL_SURFACE('',#22215,0.5);
#18791=CYLINDRICAL_SURFACE('',#22230,0.5);
#18792=CYLINDRICAL_SURFACE('',#22235,0.5);
#18793=CYLINDRICAL_SURFACE('',#22236,18.5);
#18794=CYLINDRICAL_SURFACE('',#22247,0.5);
#18795=CYLINDRICAL_SURFACE('',#22251,0.5);
#18796=CYLINDRICAL_SURFACE('',#22255,0.5);
#18797=CYLINDRICAL_SURFACE('',#22262,0.5);
#18798=CYLINDRICAL_SURFACE('',#22268,0.5);
#18799=CYLINDRICAL_SURFACE('',#22269,0.5);
#18800=CYLINDRICAL_SURFACE('',#22273,0.5);
#18801=CYLINDRICAL_SURFACE('',#22280,0.5);
#18802=CYLINDRICAL_SURFACE('',#22288,0.5);
#18803=CYLINDRICAL_SURFACE('',#22290,0.5);
#18804=CYLINDRICAL_SURFACE('',#22295,0.5);
#18805=CYLINDRICAL_SURFACE('',#22297,0.5);
#18806=CYLINDRICAL_SURFACE('',#22311,0.5);
#18807=CYLINDRICAL_SURFACE('',#22313,0.5);
#18808=CYLINDRICAL_SURFACE('',#22315,0.5);
#18809=CYLINDRICAL_SURFACE('',#22317,0.5);
#18810=CYLINDRICAL_SURFACE('',#22326,0.5);
#18811=CYLINDRICAL_SURFACE('',#22327,18.5);
#18812=CYLINDRICAL_SURFACE('',#22351,0.5);
#18813=CYLINDRICAL_SURFACE('',#22356,18.5);
#18814=CYLINDRICAL_SURFACE('',#22357,0.5);
#18815=CYLINDRICAL_SURFACE('',#22362,0.5);
#18816=CYLINDRICAL_SURFACE('',#22367,0.5);
#18817=CYLINDRICAL_SURFACE('',#22369,0.5);
#18818=CYLINDRICAL_SURFACE('',#22370,0.5);
#18819=CYLINDRICAL_SURFACE('',#22371,0.5);
#18820=CYLINDRICAL_SURFACE('',#22377,18.5);
#18821=CYLINDRICAL_SURFACE('',#22378,18.5);
#19847=ADVANCED_FACE('',(#2151),#168,.T.);
#19848=ADVANCED_FACE('',(#2152),#18771,.F.);
#19849=ADVANCED_FACE('',(#2153,#1124),#1040,.T.);
#19850=ADVANCED_FACE('',(#2154),#169,.T.);
#19851=ADVANCED_FACE('',(#2155,#1125),#1041,.T.);
#19852=ADVANCED_FACE('',(#2156),#18772,.T.);
#19853=ADVANCED_FACE('',(#2157),#1042,.F.);
#19854=ADVANCED_FACE('',(#2158),#18773,.T.);
#19855=ADVANCED_FACE('',(#2159),#18774,.T.);
#19856=ADVANCED_FACE('',(#2160),#1043,.F.);
#19857=ADVANCED_FACE('',(#2161),#18775,.T.);
#19858=ADVANCED_FACE('',(#2162),#18776,.T.);
#19859=ADVANCED_FACE('',(#2163),#1044,.F.);
#19860=ADVANCED_FACE('',(#2164),#18777,.T.);
#19861=ADVANCED_FACE('',(#2165),#170,.T.);
#19862=ADVANCED_FACE('',(#2166),#314,.T.);
#19863=ADVANCED_FACE('',(#2167),#18778,.T.);
#19864=ADVANCED_FACE('',(#2168),#315,.T.);
#19865=ADVANCED_FACE('',(#2169),#316,.T.);
#19866=ADVANCED_FACE('',(#2170),#18779,.T.);
#19867=ADVANCED_FACE('',(#2171),#844,.F.);
#19868=ADVANCED_FACE('',(#2172),#495,.T.);
#19869=ADVANCED_FACE('',(#2173),#845,.F.);
#19870=ADVANCED_FACE('',(#2174),#1045,.F.);
#19871=ADVANCED_FACE('',(#2175),#18780,.T.);
#19872=ADVANCED_FACE('',(#2176),#317,.T.);
#19873=ADVANCED_FACE('',(#2177),#1046,.T.);
#19874=ADVANCED_FACE('',(#2178),#171,.T.);
#19875=ADVANCED_FACE('',(#2179),#18781,.T.);
#19876=ADVANCED_FACE('',(#2180),#18782,.T.);
#19877=ADVANCED_FACE('',(#2181),#318,.T.);
#19878=ADVANCED_FACE('',(#2182),#319,.T.);
#19879=ADVANCED_FACE('',(#2183),#846,.F.);
#19880=ADVANCED_FACE('',(#2184),#172,.T.);
#19881=ADVANCED_FACE('',(#2185),#496,.T.);
#19882=ADVANCED_FACE('',(#2186),#173,.T.);
#19883=ADVANCED_FACE('',(#2187),#174,.T.);
#19884=ADVANCED_FACE('',(#2188),#1047,.F.);
#19885=ADVANCED_FACE('',(#2189),#320,.T.);
#19886=ADVANCED_FACE('',(#2190),#175,.T.);
#19887=ADVANCED_FACE('',(#2191),#321,.T.);
#19888=ADVANCED_FACE('',(#2192),#322,.T.);
#19889=ADVANCED_FACE('',(#2193),#323,.T.);
#19890=ADVANCED_FACE('',(#2194),#847,.F.);
#19891=ADVANCED_FACE('',(#2195),#848,.F.);
#19892=ADVANCED_FACE('',(#2196),#18783,.T.);
#19893=ADVANCED_FACE('',(#2197),#18784,.T.);
#19894=ADVANCED_FACE('',(#2198),#1048,.F.);
#19895=ADVANCED_FACE('',(#2199),#18785,.T.);
#19896=ADVANCED_FACE('',(#2200),#176,.T.);
#19897=ADVANCED_FACE('',(#2201),#1049,.F.);
#19898=ADVANCED_FACE('',(#2202),#324,.T.);
#19899=ADVANCED_FACE('',(#2203),#325,.T.);
#19900=ADVANCED_FACE('',(#2204),#18786,.T.);
#19901=ADVANCED_FACE('',(#2205),#1050,.F.);
#19902=ADVANCED_FACE('',(#2206),#18787,.T.);
#19903=ADVANCED_FACE('',(#2207),#326,.T.);
#19904=ADVANCED_FACE('',(#2208),#849,.F.);
#19905=ADVANCED_FACE('',(#2209),#18788,.T.);
#19906=ADVANCED_FACE('',(#2210),#177,.T.);
#19907=ADVANCED_FACE('',(#2211),#327,.T.);
#19908=ADVANCED_FACE('',(#2212),#1051,.F.);
#19909=ADVANCED_FACE('',(#2213),#18789,.T.);
#19910=ADVANCED_FACE('',(#2214),#1052,.T.);
#19911=ADVANCED_FACE('',(#2215),#18790,.T.);
#19912=ADVANCED_FACE('',(#2216),#328,.T.);
#19913=ADVANCED_FACE('',(#2217),#178,.T.);
#19914=ADVANCED_FACE('',(#2218),#1053,.F.);
#19915=ADVANCED_FACE('',(#2219),#179,.T.);
#19916=ADVANCED_FACE('',(#2220),#180,.T.);
#19917=ADVANCED_FACE('',(#2221),#18791,.T.);
#19918=ADVANCED_FACE('',(#2222),#181,.T.);
#19919=ADVANCED_FACE('',(#2223),#329,.T.);
#19920=ADVANCED_FACE('',(#2224),#18792,.T.);
#19921=ADVANCED_FACE('',(#2225),#18793,.F.);
#19922=ADVANCED_FACE('',(#2226),#18794,.T.);
#19923=ADVANCED_FACE('',(#2227),#182,.T.);
#19924=ADVANCED_FACE('',(#2228),#1054,.T.);
#19925=ADVANCED_FACE('',(#2229),#18795,.T.);
#19926=ADVANCED_FACE('',(#2230),#183,.T.);
#19927=ADVANCED_FACE('',(#2231),#1055,.T.);
#19928=ADVANCED_FACE('',(#2232),#18796,.T.);
#19929=ADVANCED_FACE('',(#2233),#184,.T.);
#19930=ADVANCED_FACE('',(#2234),#330,.T.);
#19931=ADVANCED_FACE('',(#2235),#18797,.T.);
#19932=ADVANCED_FACE('',(#2236),#185,.T.);
#19933=ADVANCED_FACE('',(#2237),#186,.T.);
#19934=ADVANCED_FACE('',(#2238),#187,.T.);
#19935=ADVANCED_FACE('',(#2239),#1056,.F.);
#19936=ADVANCED_FACE('',(#2240),#18798,.T.);
#19937=ADVANCED_FACE('',(#2241),#18799,.T.);
#19938=ADVANCED_FACE('',(#2242),#331,.T.);
#19939=ADVANCED_FACE('',(#2243),#18800,.T.);
#19940=ADVANCED_FACE('',(#2244),#1057,.F.);
#19941=ADVANCED_FACE('',(#2245),#188,.T.);
#19942=ADVANCED_FACE('',(#2246),#1058,.T.);
#19943=ADVANCED_FACE('',(#2247),#18801,.T.);
#19944=ADVANCED_FACE('',(#2248),#332,.T.);
#19945=ADVANCED_FACE('',(#2249),#333,.T.);
#19946=ADVANCED_FACE('',(#2250),#18802,.T.);
#19947=ADVANCED_FACE('',(#2251),#189,.T.);
#19948=ADVANCED_FACE('',(#2252),#18803,.T.);
#19949=ADVANCED_FACE('',(#2253),#1059,.F.);
#19950=ADVANCED_FACE('',(#2254),#1060,.T.);
#19951=ADVANCED_FACE('',(#2255),#18804,.T.);
#19952=ADVANCED_FACE('',(#2256),#1061,.F.);
#19953=ADVANCED_FACE('',(#2257),#18805,.T.);
#19954=ADVANCED_FACE('',(#2258),#1062,.F.);
#19955=ADVANCED_FACE('',(#2259),#190,.T.);
#19956=ADVANCED_FACE('',(#2260),#1063,.T.);
#19957=ADVANCED_FACE('',(#2261),#191,.T.);
#19958=ADVANCED_FACE('',(#2262),#497,.T.);
#19959=ADVANCED_FACE('',(#2263),#18806,.T.);
#19960=ADVANCED_FACE('',(#2264),#1064,.F.);
#19961=ADVANCED_FACE('',(#2265),#18807,.T.);
#19962=ADVANCED_FACE('',(#2266),#1065,.F.);
#19963=ADVANCED_FACE('',(#2267),#18808,.T.);
#19964=ADVANCED_FACE('',(#2268),#1066,.F.);
#19965=ADVANCED_FACE('',(#2269),#18809,.T.);
#19966=ADVANCED_FACE('',(#2270),#192,.T.);
#19967=ADVANCED_FACE('',(#2271),#334,.T.);
#19968=ADVANCED_FACE('',(#2272),#18810,.T.);
#19969=ADVANCED_FACE('',(#2273),#18811,.F.);
#19970=ADVANCED_FACE('',(#2274),#1067,.T.);
#19971=ADVANCED_FACE('',(#2275),#850,.F.);
#19972=ADVANCED_FACE('',(#2276),#1068,.F.);
#19973=ADVANCED_FACE('',(#2277),#193,.T.);
#19974=ADVANCED_FACE('',(#2278),#1069,.T.);
#19975=ADVANCED_FACE('',(#2279),#194,.T.);
#19976=ADVANCED_FACE('',(#2280),#851,.F.);
#19977=ADVANCED_FACE('',(#2281),#1070,.F.);
#19978=ADVANCED_FACE('',(#2282),#195,.T.);
#19979=ADVANCED_FACE('',(#2283),#1071,.T.);
#19980=ADVANCED_FACE('',(#2284),#196,.T.);
#19981=ADVANCED_FACE('',(#2285),#852,.F.);
#19982=ADVANCED_FACE('',(#2286),#1072,.F.);
#19983=ADVANCED_FACE('',(#2287),#1073,.T.);
#19984=ADVANCED_FACE('',(#2288),#197,.T.);
#19985=ADVANCED_FACE('',(#2289),#18812,.T.);
#19986=ADVANCED_FACE('',(#2290),#335,.T.);
#19987=ADVANCED_FACE('',(#2291),#18813,.F.);
#19988=ADVANCED_FACE('',(#2292),#18814,.T.);
#19989=ADVANCED_FACE('',(#2293),#1074,.F.);
#19990=ADVANCED_FACE('',(#2294),#198,.T.);
#19991=ADVANCED_FACE('',(#2295),#18815,.T.);
#19992=ADVANCED_FACE('',(#2296),#1075,.F.);
#19993=ADVANCED_FACE('',(#2297),#1076,.F.);
#19994=ADVANCED_FACE('',(#2298),#18816,.T.);
#19995=ADVANCED_FACE('',(#2299),#1077,.F.);
#19996=ADVANCED_FACE('',(#2300),#18817,.T.);
#19997=ADVANCED_FACE('',(#2301),#18818,.T.);
#19998=ADVANCED_FACE('',(#2302),#18819,.T.);
#19999=ADVANCED_FACE('',(#2303),#199,.T.);
#20000=ADVANCED_FACE('',(#2304),#1078,.T.);
#20001=ADVANCED_FACE('',(#2305),#1079,.F.);
#20002=ADVANCED_FACE('',(#2306),#1080,.F.);
#20003=ADVANCED_FACE('',(#2307),#18820,.F.);
#20004=ADVANCED_FACE('',(#2308),#18821,.F.);
#20005=ADVANCED_FACE('',(#2309),#1081,.F.);
#20006=ADVANCED_FACE('',(#2310),#498,.T.);
#20007=ADVANCED_FACE('',(#2311),#499,.T.);
#20018=CLOSED_SHELL('',(#19847,#19848,#19849,#19850,#19851,#19852,#19853,
#19854,#19855,#19856,#19857,#19858,#19859,#19860,#19861,#19862,#19863,#19864,
#19865,#19866,#19867,#19868,#19869,#19870,#19871,#19872,#19873,#19874,#19875,
#19876,#19877,#19878,#19879,#19880,#19881,#19882,#19883,#19884,#19885,#19886,
#19887,#19888,#19889,#19890,#19891,#19892,#19893,#19894,#19895,#19896,#19897,
#19898,#19899,#19900,#19901,#19902,#19903,#19904,#19905,#19906,#19907,#19908,
#19909,#19910,#19911,#19912,#19913,#19914,#19915,#19916,#19917,#19918,#19919,
#19920,#19921,#19922,#19923,#19924,#19925,#19926,#19927,#19928,#19929,#19930,
#19931,#19932,#19933,#19934,#19935,#19936,#19937,#19938,#19939,#19940,#19941,
#19942,#19943,#19944,#19945,#19946,#19947,#19948,#19949,#19950,#19951,#19952,
#19953,#19954,#19955,#19956,#19957,#19958,#19959,#19960,#19961,#19962,#19963,
#19964,#19965,#19966,#19967,#19968,#19969,#19970,#19971,#19972,#19973,#19974,
#19975,#19976,#19977,#19978,#19979,#19980,#19981,#19982,#19983,#19984,#19985,
#19986,#19987,#19988,#19989,#19990,#19991,#19992,#19993,#19994,#19995,#19996,
#19997,#19998,#19999,#20000,#20001,#20002,#20003,#20004,#20005,#20006,#20007));
#22041=AXIS2_PLACEMENT_3D('',#63527,#26939,#26940);
#22042=AXIS2_PLACEMENT_3D('',#63528,#26941,#26942);
#22043=AXIS2_PLACEMENT_3D('',#63530,#26943,#26944);
#22044=AXIS2_PLACEMENT_3D('',#63532,#26945,#26946);
#22045=AXIS2_PLACEMENT_3D('',#63534,#26947,#26948);
#22046=AXIS2_PLACEMENT_3D('',#63535,#26949,#26950);
#22047=AXIS2_PLACEMENT_3D('',#63536,#26951,#26952);
#22048=AXIS2_PLACEMENT_3D('',#63539,#26953,#26954);
#22049=AXIS2_PLACEMENT_3D('',#63540,#26955,#26956);
#22050=AXIS2_PLACEMENT_3D('',#63542,#26958,#26959);
#22051=AXIS2_PLACEMENT_3D('',#63547,#26961,#26962);
#22052=AXIS2_PLACEMENT_3D('',#63549,#26963,#26964);
#22053=AXIS2_PLACEMENT_3D('',#63551,#26965,#26966);
#22054=AXIS2_PLACEMENT_3D('',#63559,#26970,#26971);
#22055=AXIS2_PLACEMENT_3D('',#63561,#26972,#26973);
#22056=AXIS2_PLACEMENT_3D('',#63563,#26974,#26975);
#22057=AXIS2_PLACEMENT_3D('',#63565,#26976,#26977);
#22058=AXIS2_PLACEMENT_3D('',#63573,#26981,#26982);
#22059=AXIS2_PLACEMENT_3D('',#63575,#26983,#26984);
#22060=AXIS2_PLACEMENT_3D('',#63577,#26985,#26986);
#22061=AXIS2_PLACEMENT_3D('',#63585,#26990,#26991);
#22062=AXIS2_PLACEMENT_3D('',#63587,#26992,#26993);
#22063=AXIS2_PLACEMENT_3D('',#63589,#26994,#26995);
#22064=AXIS2_PLACEMENT_3D('',#63593,#26998,#26999);
#22065=AXIS2_PLACEMENT_3D('',#63595,#27000,#27001);
#22066=AXIS2_PLACEMENT_3D('',#63596,#27002,#27003);
#22067=AXIS2_PLACEMENT_3D('',#63597,#27004,#27005);
#22068=AXIS2_PLACEMENT_3D('',#63602,#27007,#27008);
#22069=AXIS2_PLACEMENT_3D('',#63610,#27012,#27013);
#22070=AXIS2_PLACEMENT_3D('',#63618,#27017,#27018);
#22071=AXIS2_PLACEMENT_3D('',#63620,#27019,#27020);
#22072=AXIS2_PLACEMENT_3D('',#63628,#27024,#27025);
#22073=AXIS2_PLACEMENT_3D('',#63630,#27026,#27027);
#22074=AXIS2_PLACEMENT_3D('',#63634,#27030,#27031);
#22075=AXIS2_PLACEMENT_3D('',#63636,#27032,#27033);
#22076=AXIS2_PLACEMENT_3D('',#63639,#27035,#27036);
#22077=AXIS2_PLACEMENT_3D('',#63640,#27037,#27038);
#22078=AXIS2_PLACEMENT_3D('',#63646,#27042,#27043);
#22079=AXIS2_PLACEMENT_3D('',#63647,#27044,#27045);
#22080=AXIS2_PLACEMENT_3D('',#63648,#27046,#27047);
#22081=AXIS2_PLACEMENT_3D('',#63649,#27048,#27049);
#22082=AXIS2_PLACEMENT_3D('',#63651,#27050,#27051);
#22083=AXIS2_PLACEMENT_3D('',#63654,#27053,#27054);
#22084=AXIS2_PLACEMENT_3D('',#63655,#27055,#27056);
#22085=AXIS2_PLACEMENT_3D('',#63661,#27060,#27061);
#22086=AXIS2_PLACEMENT_3D('',#63662,#27062,#27063);
#22087=AXIS2_PLACEMENT_3D('',#63663,#27064,#27065);
#22088=AXIS2_PLACEMENT_3D('',#63664,#27066,#27067);
#22089=AXIS2_PLACEMENT_3D('',#63666,#27068,#27069);
#22090=AXIS2_PLACEMENT_3D('',#63669,#27071,#27072);
#22091=AXIS2_PLACEMENT_3D('',#63670,#27073,#27074);
#22092=AXIS2_PLACEMENT_3D('',#63676,#27078,#27079);
#22093=AXIS2_PLACEMENT_3D('',#63677,#27080,#27081);
#22094=AXIS2_PLACEMENT_3D('',#63678,#27082,#27083);
#22095=AXIS2_PLACEMENT_3D('',#63679,#27084,#27085);
#22096=AXIS2_PLACEMENT_3D('',#63682,#27086,#27087);
#22097=AXIS2_PLACEMENT_3D('',#63684,#27088,#27089);
#22098=AXIS2_PLACEMENT_3D('',#63686,#27090,#27091);
#22099=AXIS2_PLACEMENT_3D('',#63687,#27092,#27093);
#22100=AXIS2_PLACEMENT_3D('',#63688,#27094,#27095);
#22101=AXIS2_PLACEMENT_3D('',#63690,#27096,#27097);
#22102=AXIS2_PLACEMENT_3D('',#63691,#27098,#27099);
#22103=AXIS2_PLACEMENT_3D('',#63692,#27100,#27101);
#22104=AXIS2_PLACEMENT_3D('',#63694,#27102,#27103);
#22105=AXIS2_PLACEMENT_3D('',#63698,#27105,#27106);
#22106=AXIS2_PLACEMENT_3D('',#63700,#27108,#27109);
#22107=AXIS2_PLACEMENT_3D('',#63702,#27110,#27111);
#22108=AXIS2_PLACEMENT_3D('',#63703,#27112,#27113);
#22109=AXIS2_PLACEMENT_3D('',#63704,#27114,#27115);
#22110=AXIS2_PLACEMENT_3D('',#63705,#27116,#27117);
#22111=AXIS2_PLACEMENT_3D('',#63706,#27118,#27119);
#22112=AXIS2_PLACEMENT_3D('',#63710,#27121,#27122);
#22113=AXIS2_PLACEMENT_3D('',#63742,#27124,#27125);
#22114=AXIS2_PLACEMENT_3D('',#63747,#27126,#27127);
#22115=AXIS2_PLACEMENT_3D('',#63753,#27128,#27129);
#22116=AXIS2_PLACEMENT_3D('',#63783,#27130,#27131);
#22117=AXIS2_PLACEMENT_3D('',#63784,#27132,#27133);
#22118=AXIS2_PLACEMENT_3D('',#63795,#27137,#27138);
#22119=AXIS2_PLACEMENT_3D('',#63814,#27140,#27141);
#22120=AXIS2_PLACEMENT_3D('',#63815,#27142,#27143);
#22121=AXIS2_PLACEMENT_3D('',#63816,#27144,#27145);
#22122=AXIS2_PLACEMENT_3D('',#63817,#27146,#27147);
#22123=AXIS2_PLACEMENT_3D('',#63818,#27148,#27149);
#22124=AXIS2_PLACEMENT_3D('',#63819,#27150,#27151);
#22125=AXIS2_PLACEMENT_3D('',#63820,#27152,#27153);
#22126=AXIS2_PLACEMENT_3D('',#63822,#27154,#27155);
#22127=AXIS2_PLACEMENT_3D('',#63823,#27156,#27157);
#22128=AXIS2_PLACEMENT_3D('',#63824,#27158,#27159);
#22129=AXIS2_PLACEMENT_3D('',#63827,#27160,#27161);
#22130=AXIS2_PLACEMENT_3D('',#63831,#27163,#27164);
#22131=AXIS2_PLACEMENT_3D('',#63835,#27166,#27167);
#22132=AXIS2_PLACEMENT_3D('',#63839,#27169,#27170);
#22133=AXIS2_PLACEMENT_3D('',#63843,#27172,#27173);
#22134=AXIS2_PLACEMENT_3D('',#63847,#27175,#27176);
#22135=AXIS2_PLACEMENT_3D('',#63851,#27178,#27179);
#22136=AXIS2_PLACEMENT_3D('',#63855,#27181,#27182);
#22137=AXIS2_PLACEMENT_3D('',#63857,#27184,#27185);
#22138=AXIS2_PLACEMENT_3D('',#63858,#27186,#27187);
#22139=AXIS2_PLACEMENT_3D('',#63859,#27188,#27189);
#22140=AXIS2_PLACEMENT_3D('',#63862,#27190,#27191);
#22141=AXIS2_PLACEMENT_3D('',#63865,#27193,#27194);
#22142=AXIS2_PLACEMENT_3D('',#63880,#27195,#27196);
#22143=AXIS2_PLACEMENT_3D('',#63882,#27197,#27198);
#22144=AXIS2_PLACEMENT_3D('',#63883,#27199,#27200);
#22145=AXIS2_PLACEMENT_3D('',#63884,#27201,#27202);
#22146=AXIS2_PLACEMENT_3D('',#63887,#27203,#27204);
#22147=AXIS2_PLACEMENT_3D('',#63889,#27205,#27206);
#22148=AXIS2_PLACEMENT_3D('',#63890,#27207,#27208);
#22149=AXIS2_PLACEMENT_3D('',#63923,#27209,#27210);
#22150=AXIS2_PLACEMENT_3D('',#63925,#27211,#27212);
#22151=AXIS2_PLACEMENT_3D('',#63926,#27213,#27214);
#22152=AXIS2_PLACEMENT_3D('',#63927,#27215,#27216);
#22153=AXIS2_PLACEMENT_3D('',#63929,#27217,#27218);
#22154=AXIS2_PLACEMENT_3D('',#63934,#27219,#27220);
#22155=AXIS2_PLACEMENT_3D('',#63936,#27221,#27222);
#22156=AXIS2_PLACEMENT_3D('',#63937,#27223,#27224);
#22157=AXIS2_PLACEMENT_3D('',#63938,#27225,#27226);
#22158=AXIS2_PLACEMENT_3D('',#63954,#27227,#27228);
#22159=AXIS2_PLACEMENT_3D('',#63955,#27229,#27230);
#22160=AXIS2_PLACEMENT_3D('',#63957,#27231,#27232);
#22161=AXIS2_PLACEMENT_3D('',#63961,#27234,#27235);
#22162=AXIS2_PLACEMENT_3D('',#63963,#27237,#27238);
#22163=AXIS2_PLACEMENT_3D('',#63966,#27239,#27240);
#22164=AXIS2_PLACEMENT_3D('',#63968,#27241,#27242);
#22165=AXIS2_PLACEMENT_3D('',#63969,#27243,#27244);
#22166=AXIS2_PLACEMENT_3D('',#63970,#27245,#27246);
#22167=AXIS2_PLACEMENT_3D('',#63972,#27247,#27248);
#22168=AXIS2_PLACEMENT_3D('',#63974,#27249,#27250);
#22169=AXIS2_PLACEMENT_3D('',#63975,#27251,#27252);
#22170=AXIS2_PLACEMENT_3D('',#63976,#27253,#27254);
#22171=AXIS2_PLACEMENT_3D('',#63978,#27255,#27256);
#22172=AXIS2_PLACEMENT_3D('',#63979,#27257,#27258);
#22173=AXIS2_PLACEMENT_3D('',#63980,#27259,#27260);
#22174=AXIS2_PLACEMENT_3D('',#63982,#27261,#27262);
#22175=AXIS2_PLACEMENT_3D('',#63983,#27263,#27264);
#22176=AXIS2_PLACEMENT_3D('',#63984,#27265,#27266);
#22177=AXIS2_PLACEMENT_3D('',#63987,#27267,#27268);
#22178=AXIS2_PLACEMENT_3D('',#63989,#27269,#27270);
#22179=AXIS2_PLACEMENT_3D('',#63990,#27271,#27272);
#22180=AXIS2_PLACEMENT_3D('',#64055,#27273,#27274);
#22181=AXIS2_PLACEMENT_3D('',#64072,#27275,#27276);
#22182=AXIS2_PLACEMENT_3D('',#64074,#27278,#27279);
#22183=AXIS2_PLACEMENT_3D('',#64076,#27281,#27282);
#22184=AXIS2_PLACEMENT_3D('',#64085,#27285,#27286);
#22185=AXIS2_PLACEMENT_3D('',#64088,#27288,#27289);
#22186=AXIS2_PLACEMENT_3D('',#64089,#27290,#27291);
#22187=AXIS2_PLACEMENT_3D('',#64091,#27292,#27293);
#22188=AXIS2_PLACEMENT_3D('',#64106,#27294,#27295);
#22189=AXIS2_PLACEMENT_3D('',#64108,#27296,#27297);
#22190=AXIS2_PLACEMENT_3D('',#64111,#27299,#27300);
#22191=AXIS2_PLACEMENT_3D('',#64112,#27301,#27302);
#22192=AXIS2_PLACEMENT_3D('',#64113,#27303,#27304);
#22193=AXIS2_PLACEMENT_3D('',#64114,#27305,#27306);
#22194=AXIS2_PLACEMENT_3D('',#64116,#27307,#27308);
#22195=AXIS2_PLACEMENT_3D('',#64117,#27309,#27310);
#22196=AXIS2_PLACEMENT_3D('',#64118,#27311,#27312);
#22197=AXIS2_PLACEMENT_3D('',#64135,#27315,#27316);
#22198=AXIS2_PLACEMENT_3D('',#64144,#27319,#27320);
#22199=AXIS2_PLACEMENT_3D('',#64162,#27321,#27322);
#22200=AXIS2_PLACEMENT_3D('',#64163,#27323,#27324);
#22201=AXIS2_PLACEMENT_3D('',#64165,#27325,#27326);
#22202=AXIS2_PLACEMENT_3D('',#64166,#27327,#27328);
#22203=AXIS2_PLACEMENT_3D('',#64192,#27329,#27330);
#22204=AXIS2_PLACEMENT_3D('',#64197,#27331,#27332);
#22205=AXIS2_PLACEMENT_3D('',#64198,#27333,#27334);
#22206=AXIS2_PLACEMENT_3D('',#64202,#27336,#27337);
#22207=AXIS2_PLACEMENT_3D('',#64217,#27338,#27339);
#22208=AXIS2_PLACEMENT_3D('',#64218,#27340,#27341);
#22209=AXIS2_PLACEMENT_3D('',#64219,#27342,#27343);
#22210=AXIS2_PLACEMENT_3D('',#64220,#27344,#27345);
#22211=AXIS2_PLACEMENT_3D('',#64231,#27349,#27350);
#22212=AXIS2_PLACEMENT_3D('',#64234,#27352,#27353);
#22213=AXIS2_PLACEMENT_3D('',#64235,#27354,#27355);
#22214=AXIS2_PLACEMENT_3D('',#64238,#27357,#27358);
#22215=AXIS2_PLACEMENT_3D('',#64239,#27359,#27360);
#22216=AXIS2_PLACEMENT_3D('',#64242,#27362,#27363);
#22217=AXIS2_PLACEMENT_3D('',#64243,#27364,#27365);
#22218=AXIS2_PLACEMENT_3D('',#64245,#27366,#27367);
#22219=AXIS2_PLACEMENT_3D('',#64246,#27368,#27369);
#22220=AXIS2_PLACEMENT_3D('',#64247,#27370,#27371);
#22221=AXIS2_PLACEMENT_3D('',#64263,#27372,#27373);
#22222=AXIS2_PLACEMENT_3D('',#64264,#27374,#27375);
#22223=AXIS2_PLACEMENT_3D('',#64266,#27376,#27377);
#22224=AXIS2_PLACEMENT_3D('',#64270,#27379,#27380);
#22225=AXIS2_PLACEMENT_3D('',#64272,#27382,#27383);
#22226=AXIS2_PLACEMENT_3D('',#64288,#27384,#27385);
#22227=AXIS2_PLACEMENT_3D('',#64310,#27386,#27387);
#22228=AXIS2_PLACEMENT_3D('',#64312,#27388,#27389);
#22229=AXIS2_PLACEMENT_3D('',#64313,#27390,#27391);
#22230=AXIS2_PLACEMENT_3D('',#64314,#27392,#27393);
#22231=AXIS2_PLACEMENT_3D('',#64331,#27396,#27397);
#22232=AXIS2_PLACEMENT_3D('',#64345,#27398,#27399);
#22233=AXIS2_PLACEMENT_3D('',#64350,#27400,#27401);
#22234=AXIS2_PLACEMENT_3D('',#64351,#27402,#27403);
#22235=AXIS2_PLACEMENT_3D('',#64352,#27404,#27405);
#22236=AXIS2_PLACEMENT_3D('',#64367,#27407,#27408);
#22237=AXIS2_PLACEMENT_3D('',#64373,#27411,#27412);
#22238=AXIS2_PLACEMENT_3D('',#64378,#27415,#27416);
#22239=AXIS2_PLACEMENT_3D('',#64383,#27419,#27420);
#22240=AXIS2_PLACEMENT_3D('',#64385,#27422,#27423);
#22241=AXIS2_PLACEMENT_3D('',#64386,#27424,#27425);
#22242=AXIS2_PLACEMENT_3D('',#64390,#27427,#27428);
#22243=AXIS2_PLACEMENT_3D('',#64395,#27431,#27432);
#22244=AXIS2_PLACEMENT_3D('',#64398,#27434,#27435);
#22245=AXIS2_PLACEMENT_3D('',#64402,#27437,#27438);
#22246=AXIS2_PLACEMENT_3D('',#64406,#27441,#27442);
#22247=AXIS2_PLACEMENT_3D('',#64407,#27443,#27444);
#22248=AXIS2_PLACEMENT_3D('',#64422,#27446,#27447);
#22249=AXIS2_PLACEMENT_3D('',#64442,#27448,#27449);
#22250=AXIS2_PLACEMENT_3D('',#64447,#27450,#27451);
#22251=AXIS2_PLACEMENT_3D('',#64453,#27455,#27456);
#22252=AXIS2_PLACEMENT_3D('',#64468,#27458,#27459);
#22253=AXIS2_PLACEMENT_3D('',#64488,#27460,#27461);
#22254=AXIS2_PLACEMENT_3D('',#64493,#27462,#27463);
#22255=AXIS2_PLACEMENT_3D('',#64499,#27467,#27468);
#22256=AXIS2_PLACEMENT_3D('',#64512,#27469,#27470);
#22257=AXIS2_PLACEMENT_3D('',#64514,#27471,#27472);
#22258=AXIS2_PLACEMENT_3D('',#64516,#27473,#27474);
#22259=AXIS2_PLACEMENT_3D('',#64534,#27475,#27476);
#22260=AXIS2_PLACEMENT_3D('',#64536,#27477,#27478);
#22261=AXIS2_PLACEMENT_3D('',#64537,#27479,#27480);
#22262=AXIS2_PLACEMENT_3D('',#64538,#27481,#27482);
#22263=AXIS2_PLACEMENT_3D('',#64553,#27484,#27485);
#22264=AXIS2_PLACEMENT_3D('',#64558,#27486,#27487);
#22265=AXIS2_PLACEMENT_3D('',#64559,#27488,#27489);
#22266=AXIS2_PLACEMENT_3D('',#64560,#27490,#27491);
#22267=AXIS2_PLACEMENT_3D('',#64561,#27492,#27493);
#22268=AXIS2_PLACEMENT_3D('',#64562,#27494,#27495);
#22269=AXIS2_PLACEMENT_3D('',#64564,#27497,#27498);
#22270=AXIS2_PLACEMENT_3D('',#64568,#27500,#27501);
#22271=AXIS2_PLACEMENT_3D('',#64570,#27503,#27504);
#22272=AXIS2_PLACEMENT_3D('',#64592,#27505,#27506);
#22273=AXIS2_PLACEMENT_3D('',#64593,#27507,#27508);
#22274=AXIS2_PLACEMENT_3D('',#64595,#27510,#27511);
#22275=AXIS2_PLACEMENT_3D('',#64596,#27512,#27513);
#22276=AXIS2_PLACEMENT_3D('',#64597,#27514,#27515);
#22277=AXIS2_PLACEMENT_3D('',#64598,#27516,#27517);
#22278=AXIS2_PLACEMENT_3D('',#64599,#27518,#27519);
#22279=AXIS2_PLACEMENT_3D('',#64602,#27521,#27522);
#22280=AXIS2_PLACEMENT_3D('',#64603,#27523,#27524);
#22281=AXIS2_PLACEMENT_3D('',#64606,#27526,#27527);
#22282=AXIS2_PLACEMENT_3D('',#64607,#27528,#27529);
#22283=AXIS2_PLACEMENT_3D('',#64608,#27530,#27531);
#22284=AXIS2_PLACEMENT_3D('',#64609,#27532,#27533);
#22285=AXIS2_PLACEMENT_3D('',#64610,#27534,#27535);
#22286=AXIS2_PLACEMENT_3D('',#64611,#27536,#27537);
#22287=AXIS2_PLACEMENT_3D('',#64612,#27538,#27539);
#22288=AXIS2_PLACEMENT_3D('',#64613,#27540,#27541);
#22289=AXIS2_PLACEMENT_3D('',#64614,#27542,#27543);
#22290=AXIS2_PLACEMENT_3D('',#64615,#27544,#27545);
#22291=AXIS2_PLACEMENT_3D('',#64617,#27547,#27548);
#22292=AXIS2_PLACEMENT_3D('',#64618,#27549,#27550);
#22293=AXIS2_PLACEMENT_3D('',#64620,#27551,#27552);
#22294=AXIS2_PLACEMENT_3D('',#64622,#27553,#27554);
#22295=AXIS2_PLACEMENT_3D('',#64624,#27556,#27557);
#22296=AXIS2_PLACEMENT_3D('',#64638,#27559,#27560);
#22297=AXIS2_PLACEMENT_3D('',#64639,#27561,#27562);
#22298=AXIS2_PLACEMENT_3D('',#64654,#27564,#27565);
#22299=AXIS2_PLACEMENT_3D('',#64751,#27570,#27571);
#22300=AXIS2_PLACEMENT_3D('',#64758,#27572,#27573);
#22301=AXIS2_PLACEMENT_3D('',#64771,#27574,#27575);
#22302=AXIS2_PLACEMENT_3D('',#64775,#27578,#27579);
#22303=AXIS2_PLACEMENT_3D('',#64778,#27580,#27581);
#22304=AXIS2_PLACEMENT_3D('',#64779,#27582,#27583);
#22305=AXIS2_PLACEMENT_3D('',#64780,#27584,#27585);
#22306=AXIS2_PLACEMENT_3D('',#64781,#27586,#27587);
#22307=AXIS2_PLACEMENT_3D('',#64788,#27588,#27589);
#22308=AXIS2_PLACEMENT_3D('',#64791,#27591,#27592);
#22309=AXIS2_PLACEMENT_3D('',#64805,#27593,#27594);
#22310=AXIS2_PLACEMENT_3D('',#64816,#27595,#27596);
#22311=AXIS2_PLACEMENT_3D('',#64825,#27597,#27598);
#22312=AXIS2_PLACEMENT_3D('',#64827,#27600,#27601);
#22313=AXIS2_PLACEMENT_3D('',#64912,#27605,#27606);
#22314=AXIS2_PLACEMENT_3D('',#64914,#27608,#27609);
#22315=AXIS2_PLACEMENT_3D('',#64999,#27613,#27614);
#22316=AXIS2_PLACEMENT_3D('',#65001,#27616,#27617);
#22317=AXIS2_PLACEMENT_3D('',#65086,#27621,#27622);
#22318=AXIS2_PLACEMENT_3D('',#65098,#27624,#27625);
#22319=AXIS2_PLACEMENT_3D('',#65101,#27627,#27628);
#22320=AXIS2_PLACEMENT_3D('',#65102,#27629,#27630);
#22321=AXIS2_PLACEMENT_3D('',#65104,#27631,#27632);
#22322=AXIS2_PLACEMENT_3D('',#65105,#27633,#27634);
#22323=AXIS2_PLACEMENT_3D('',#65106,#27635,#27636);
#22324=AXIS2_PLACEMENT_3D('',#65107,#27637,#27638);
#22325=AXIS2_PLACEMENT_3D('',#65108,#27639,#27640);
#22326=AXIS2_PLACEMENT_3D('',#65109,#27641,#27642);
#22327=AXIS2_PLACEMENT_3D('',#65112,#27645,#27646);
#22328=AXIS2_PLACEMENT_3D('',#65113,#27647,#27648);
#22329=AXIS2_PLACEMENT_3D('',#65114,#27649,#27650);
#22330=AXIS2_PLACEMENT_3D('',#65209,#27651,#27652);
#22331=AXIS2_PLACEMENT_3D('',#65211,#27654,#27655);
#22332=AXIS2_PLACEMENT_3D('',#65219,#27656,#27657);
#22333=AXIS2_PLACEMENT_3D('',#65220,#27658,#27659);
#22334=AXIS2_PLACEMENT_3D('',#65223,#27661,#27662);
#22335=AXIS2_PLACEMENT_3D('',#65224,#27663,#27664);
#22336=AXIS2_PLACEMENT_3D('',#65226,#27665,#27666);
#22337=AXIS2_PLACEMENT_3D('',#65269,#27667,#27668);
#22338=AXIS2_PLACEMENT_3D('',#65270,#27669,#27670);
#22339=AXIS2_PLACEMENT_3D('',#65271,#27671,#27672);
#22340=AXIS2_PLACEMENT_3D('',#65272,#27673,#27674);
#22341=AXIS2_PLACEMENT_3D('',#65273,#27675,#27676);
#22342=AXIS2_PLACEMENT_3D('',#65274,#27677,#27678);
#22343=AXIS2_PLACEMENT_3D('',#65275,#27679,#27680);
#22344=AXIS2_PLACEMENT_3D('',#65370,#27681,#27682);
#22345=AXIS2_PLACEMENT_3D('',#65372,#27684,#27685);
#22346=AXIS2_PLACEMENT_3D('',#65377,#27687,#27688);
#22347=AXIS2_PLACEMENT_3D('',#65380,#27690,#27691);
#22348=AXIS2_PLACEMENT_3D('',#65381,#27692,#27693);
#22349=AXIS2_PLACEMENT_3D('',#65394,#27694,#27695);
#22350=AXIS2_PLACEMENT_3D('',#65395,#27696,#27697);
#22351=AXIS2_PLACEMENT_3D('',#65396,#27698,#27699);
#22352=AXIS2_PLACEMENT_3D('',#65405,#27700,#27701);
#22353=AXIS2_PLACEMENT_3D('',#65408,#27703,#27704);
#22354=AXIS2_PLACEMENT_3D('',#65409,#27705,#27706);
#22355=AXIS2_PLACEMENT_3D('',#65410,#27707,#27708);
#22356=AXIS2_PLACEMENT_3D('',#65411,#27709,#27710);
#22357=AXIS2_PLACEMENT_3D('',#65414,#27713,#27714);
#22358=AXIS2_PLACEMENT_3D('',#65416,#27716,#27717);
#22359=AXIS2_PLACEMENT_3D('',#65428,#27721,#27722);
#22360=AXIS2_PLACEMENT_3D('',#65431,#27724,#27725);
#22361=AXIS2_PLACEMENT_3D('',#65432,#27726,#27727);
#22362=AXIS2_PLACEMENT_3D('',#65455,#27728,#27729);
#22363=AXIS2_PLACEMENT_3D('',#65457,#27731,#27732);
#22364=AXIS2_PLACEMENT_3D('',#65459,#27733,#27734);
#22365=AXIS2_PLACEMENT_3D('',#65462,#27736,#27737);
#22366=AXIS2_PLACEMENT_3D('',#65473,#27741,#27742);
#22367=AXIS2_PLACEMENT_3D('',#65475,#27744,#27745);
#22368=AXIS2_PLACEMENT_3D('',#65477,#27747,#27748);
#22369=AXIS2_PLACEMENT_3D('',#65479,#27750,#27751);
#22370=AXIS2_PLACEMENT_3D('',#65480,#27752,#27753);
#22371=AXIS2_PLACEMENT_3D('',#65493,#27754,#27755);
#22372=AXIS2_PLACEMENT_3D('',#65506,#27756,#27757);
#22373=AXIS2_PLACEMENT_3D('',#65507,#27758,#27759);
#22374=AXIS2_PLACEMENT_3D('',#65508,#27760,#27761);
#22375=AXIS2_PLACEMENT_3D('',#65509,#27762,#27763);
#22376=AXIS2_PLACEMENT_3D('',#65510,#27764,#27765);
#22377=AXIS2_PLACEMENT_3D('',#65512,#27767,#27768);
#22378=AXIS2_PLACEMENT_3D('',#65513,#27769,#27770);
#22379=AXIS2_PLACEMENT_3D('',#65514,#27771,#27772);
#22380=AXIS2_PLACEMENT_3D('',#65515,#27773,#27774);
#22381=AXIS2_PLACEMENT_3D('',#65516,#27775,#27776);
#26939=DIRECTION('axis',(0.,0.,1.));
#26940=DIRECTION('refdir',(1.,0.,0.));
#26941=DIRECTION('center_axis',(1.,0.,0.));
#26942=DIRECTION('ref_axis',(0.,0.,-1.));
#26943=DIRECTION('center_axis',(-1.,0.,0.));
#26944=DIRECTION('ref_axis',(0.,-1.,1.83697019872103E-16));
#26945=DIRECTION('center_axis',(0.,-1.,-1.22464679914735E-16));
#26946=DIRECTION('ref_axis',(0.,-1.22464679914735E-16,1.));
#26947=DIRECTION('center_axis',(1.,0.,0.));
#26948=DIRECTION('ref_axis',(0.,-1.,1.83697019872103E-16));
#26949=DIRECTION('center_axis',(1.,0.,0.));
#26950=DIRECTION('ref_axis',(0.,-1.,1.83697019872103E-16));
#26951=DIRECTION('center_axis',(1.,0.,0.));
#26952=DIRECTION('ref_axis',(0.,1.,0.));
#26953=DIRECTION('center_axis',(-1.,0.,0.));
#26954=DIRECTION('ref_axis',(0.,-1.,1.83697019872103E-16));
#26955=DIRECTION('center_axis',(-1.,0.,0.));
#26956=DIRECTION('ref_axis',(0.,-1.,1.83697019872103E-16));
#26957=DIRECTION('',(-1.,0.,0.));
#26958=DIRECTION('center_axis',(-1.,0.,0.));
#26959=DIRECTION('ref_axis',(0.,0.,1.));
#26960=DIRECTION('',(0.,0.707106781186548,-0.707106781186548));
#26961=DIRECTION('center_axis',(1.,0.,0.));
#26962=DIRECTION('ref_axis',(0.,0.0791961191078487,0.996859054590094));
#26963=DIRECTION('center_axis',(1.,0.,0.));
#26964=DIRECTION('ref_axis',(0.,0.,-1.));
#26965=DIRECTION('center_axis',(1.,0.,0.));
#26966=DIRECTION('ref_axis',(0.,-0.0791961191078487,0.996859054590094));
#26967=DIRECTION('',(0.,0.707106781186547,0.707106781186548));
#26968=DIRECTION('',(0.,0.707106781186548,-0.707106781186548));
#26969=DIRECTION('',(0.,-0.707106781186548,-0.707106781186548));
#26970=DIRECTION('center_axis',(1.,0.,0.));
#26971=DIRECTION('ref_axis',(0.,0.996859054590094,-0.0791961191078487));
#26972=DIRECTION('center_axis',(1.,0.,0.));
#26973=DIRECTION('ref_axis',(0.,0.,-1.));
#26974=DIRECTION('center_axis',(1.,0.,0.));
#26975=DIRECTION('ref_axis',(0.,0.,-1.));
#26976=DIRECTION('center_axis',(1.,0.,0.));
#26977=DIRECTION('ref_axis',(0.,0.996859054590094,0.0791961191078482));
#26978=DIRECTION('',(0.,0.707106781186548,-0.707106781186547));
#26979=DIRECTION('',(0.,-0.707106781186548,-0.707106781186548));
#26980=DIRECTION('',(0.,-0.707106781186548,0.707106781186548));
#26981=DIRECTION('center_axis',(1.,0.,0.));
#26982=DIRECTION('ref_axis',(0.,-0.0791961191078482,-0.996859054590094));
#26983=DIRECTION('center_axis',(1.,0.,0.));
#26984=DIRECTION('ref_axis',(0.,0.,-1.));
#26985=DIRECTION('center_axis',(1.,0.,0.));
#26986=DIRECTION('ref_axis',(0.,0.0791961191078487,-0.996859054590094));
#26987=DIRECTION('',(0.,-0.707106781186548,-0.707106781186548));
#26988=DIRECTION('',(0.,-0.707106781186548,0.707106781186548));
#26989=DIRECTION('',(0.,0.707106781186548,0.707106781186548));
#26990=DIRECTION('center_axis',(1.,0.,0.));
#26991=DIRECTION('ref_axis',(0.,-0.996859054590094,0.0791961191078482));
#26992=DIRECTION('center_axis',(1.,0.,0.));
#26993=DIRECTION('ref_axis',(0.,0.,-1.));
#26994=DIRECTION('center_axis',(1.,0.,0.));
#26995=DIRECTION('ref_axis',(0.,-0.996859054590094,-0.0791961191078487));
#26996=DIRECTION('',(0.,-0.707106781186548,0.707106781186548));
#26997=DIRECTION('',(0.,0.707106781186547,0.707106781186547));
#26998=DIRECTION('center_axis',(1.,0.,0.));
#26999=DIRECTION('ref_axis',(0.,0.,-1.));
#27000=DIRECTION('center_axis',(0.,-1.,-1.22464679914735E-16));
#27001=DIRECTION('ref_axis',(0.,-1.22464679914735E-16,1.));
#27002=DIRECTION('center_axis',(1.,0.,0.));
#27003=DIRECTION('ref_axis',(0.,-1.,1.83697019872103E-16));
#27004=DIRECTION('center_axis',(1.,0.,0.));
#27005=DIRECTION('ref_axis',(0.,0.,-1.));
#27006=DIRECTION('',(0.,0.707106781186548,-0.707106781186548));
#27007=DIRECTION('center_axis',(1.,0.,0.));
#27008=DIRECTION('ref_axis',(0.,0.,-1.));
#27009=DIRECTION('',(0.,-0.707106781186548,-0.707106781186548));
#27010=DIRECTION('',(0.,0.707106781186548,-0.707106781186548));
#27011=DIRECTION('',(0.,0.707106781186548,0.707106781186548));
#27012=DIRECTION('center_axis',(1.,0.,0.));
#27013=DIRECTION('ref_axis',(0.,0.,-1.));
#27014=DIRECTION('',(0.,0.707106781186548,-0.707106781186548));
#27015=DIRECTION('',(0.,0.707106781186548,0.707106781186548));
#27016=DIRECTION('',(0.,-0.707106781186548,0.707106781186547));
#27017=DIRECTION('center_axis',(1.,0.,0.));
#27018=DIRECTION('ref_axis',(0.,0.,-1.));
#27019=DIRECTION('center_axis',(-1.,0.,0.));
#27020=DIRECTION('ref_axis',(0.,0.996859054590094,-0.0791961191078487));
#27021=DIRECTION('',(0.,0.707106781186548,0.707106781186548));
#27022=DIRECTION('',(0.,-0.707106781186548,0.707106781186548));
#27023=DIRECTION('',(0.,-0.707106781186547,-0.707106781186548));
#27024=DIRECTION('center_axis',(-1.,0.,0.));
#27025=DIRECTION('ref_axis',(0.,-0.0791961191078487,0.996859054590094));
#27026=DIRECTION('center_axis',(1.,0.,0.));
#27027=DIRECTION('ref_axis',(0.,0.,-1.));
#27028=DIRECTION('',(0.,-0.707106781186548,0.707106781186548));
#27029=DIRECTION('',(0.,-0.707106781186548,-0.707106781186548));
#27030=DIRECTION('center_axis',(0.,-0.707106781186548,-0.707106781186548));
#27031=DIRECTION('ref_axis',(-0.707106781186547,0.5,-0.5));
#27032=DIRECTION('center_axis',(0.,0.707106781186548,0.707106781186548));
#27033=DIRECTION('ref_axis',(-0.707106781186547,0.5,-0.5));
#27034=DIRECTION('',(0.,-0.707106781186547,-0.707106781186547));
#27035=DIRECTION('center_axis',(0.,-0.707106781186548,-0.707106781186548));
#27036=DIRECTION('ref_axis',(-0.707106781186547,0.5,-0.5));
#27037=DIRECTION('center_axis',(0.,-0.707106781186548,0.707106781186548));
#27038=DIRECTION('ref_axis',(0.,-0.707106781186548,-0.707106781186548));
#27039=DIRECTION('',(1.,0.,0.));
#27040=DIRECTION('',(0.,0.707106781186548,0.707106781186548));
#27041=DIRECTION('',(1.,0.,0.));
#27042=DIRECTION('center_axis',(0.,0.707106781186548,0.707106781186548));
#27043=DIRECTION('ref_axis',(0.707106781186545,0.500000000000005,-0.499999999999999));
#27044=DIRECTION('center_axis',(0.,-0.707106781186548,-0.707106781186548));
#27045=DIRECTION('ref_axis',(0.707106781186545,0.500000000000005,-0.499999999999999));
#27046=DIRECTION('center_axis',(0.,0.707106781186548,0.707106781186548));
#27047=DIRECTION('ref_axis',(0.707106781186545,0.500000000000005,-0.499999999999999));
#27048=DIRECTION('center_axis',(0.,0.707106781186548,-0.707106781186548));
#27049=DIRECTION('ref_axis',(-0.707106781186547,0.5,0.5));
#27050=DIRECTION('center_axis',(0.,-0.707106781186548,0.707106781186548));
#27051=DIRECTION('ref_axis',(-0.707106781186547,0.5,0.5));
#27052=DIRECTION('',(0.,0.707106781186548,-0.707106781186548));
#27053=DIRECTION('center_axis',(0.,0.707106781186548,-0.707106781186548));
#27054=DIRECTION('ref_axis',(-0.707106781186547,0.5,0.5));
#27055=DIRECTION('center_axis',(0.,-0.707106781186548,-0.707106781186548));
#27056=DIRECTION('ref_axis',(0.,0.707106781186548,-0.707106781186548));
#27057=DIRECTION('',(1.,0.,0.));
#27058=DIRECTION('',(0.,-0.707106781186548,0.707106781186548));
#27059=DIRECTION('',(1.,0.,0.));
#27060=DIRECTION('center_axis',(0.,-0.707106781186548,0.707106781186548));
#27061=DIRECTION('ref_axis',(0.707106781186543,0.500000000000004,0.500000000000004));
#27062=DIRECTION('center_axis',(0.,0.707106781186548,-0.707106781186548));
#27063=DIRECTION('ref_axis',(0.707106781186543,0.500000000000004,0.500000000000004));
#27064=DIRECTION('center_axis',(0.,-0.707106781186548,0.707106781186548));
#27065=DIRECTION('ref_axis',(0.707106781186543,0.500000000000004,0.500000000000004));
#27066=DIRECTION('center_axis',(0.,0.707106781186548,0.707106781186548));
#27067=DIRECTION('ref_axis',(-0.707106781186547,-0.5,0.5));
#27068=DIRECTION('center_axis',(0.,-0.707106781186547,-0.707106781186548));
#27069=DIRECTION('ref_axis',(-0.707106781186547,-0.5,0.5));
#27070=DIRECTION('',(0.,0.707106781186548,0.707106781186548));
#27071=DIRECTION('center_axis',(0.,0.707106781186548,0.707106781186548));
#27072=DIRECTION('ref_axis',(-0.707106781186547,-0.5,0.5));
#27073=DIRECTION('center_axis',(0.,0.707106781186548,-0.707106781186548));
#27074=DIRECTION('ref_axis',(0.,0.707106781186548,0.707106781186548));
#27075=DIRECTION('',(1.,0.,0.));
#27076=DIRECTION('',(0.,-0.707106781186548,-0.707106781186548));
#27077=DIRECTION('',(1.,0.,0.));
#27078=DIRECTION('center_axis',(0.,-0.707106781186548,-0.707106781186548));
#27079=DIRECTION('ref_axis',(0.707106781186547,-0.5,0.5));
#27080=DIRECTION('center_axis',(0.,0.707106781186548,0.707106781186548));
#27081=DIRECTION('ref_axis',(0.707106781186547,-0.5,0.5));
#27082=DIRECTION('center_axis',(0.,-0.707106781186547,-0.707106781186548));
#27083=DIRECTION('ref_axis',(0.707106781186547,-0.5,0.5));
#27084=DIRECTION('center_axis',(1.,0.,0.));
#27085=DIRECTION('ref_axis',(0.,0.,-1.));
#27086=DIRECTION('center_axis',(0.,0.197113341951552,0.980380706881103));
#27087=DIRECTION('ref_axis',(-1.,0.,0.));
#27088=DIRECTION('center_axis',(-1.,0.,0.));
#27089=DIRECTION('ref_axis',(0.,-0.707106781185558,0.707106781187537));
#27090=DIRECTION('center_axis',(-4.6165181164541E-10,-0.980380706790106,
-0.197113342404141));
#27091=DIRECTION('ref_axis',(-0.707106782908637,-0.139380180416835,0.693233844291786));
#27092=DIRECTION('center_axis',(1.,0.,0.));
#27093=DIRECTION('ref_axis',(0.,-0.707106781185558,0.707106781187537));
#27094=DIRECTION('center_axis',(0.,0.,1.));
#27095=DIRECTION('ref_axis',(-0.772461049429073,0.635062144293718,0.));
#27096=DIRECTION('center_axis',(-0.700067241886871,-1.1325494929406E-16,
-0.714076926414031));
#27097=DIRECTION('ref_axis',(-0.707106781186542,-0.139380180748398,0.69323384598168));
#27098=DIRECTION('center_axis',(0.,1.58603289232165E-16,1.));
#27099=DIRECTION('ref_axis',(-0.707106781186548,0.707106781186547,0.));
#27100=DIRECTION('center_axis',(0.,-1.,1.58603289232165E-16));
#27101=DIRECTION('ref_axis',(-0.707106781186548,0.,-0.707106781186548));
#27102=DIRECTION('center_axis',(0.,1.,-4.44089209850062E-15));
#27103=DIRECTION('ref_axis',(9.00728158725882E-9,-4.44089209850062E-15,
-1.));
#27104=DIRECTION('',(0.,1.,-1.58603289232165E-16));
#27105=DIRECTION('center_axis',(9.86076131526263E-30,-1.,-8.88178419700124E-15));
#27106=DIRECTION('ref_axis',(-1.,0.,-1.11022302462516E-15));
#27107=DIRECTION('',(0.,-1.,1.58603289232165E-16));
#27108=DIRECTION('center_axis',(-0.33661593132292,-0.848909755674506,-0.407482443180382));
#27109=DIRECTION('ref_axis',(-0.540654873563244,0.52853781957458,-0.654476952208144));
#27110=DIRECTION('center_axis',(0.,-0.210526315789474,-0.9775881905793));
#27111=DIRECTION('ref_axis',(0.,-0.9775881905793,0.210526315789474));
#27112=DIRECTION('center_axis',(-1.,0.,0.));
#27113=DIRECTION('ref_axis',(0.,0.62828086243754,-0.777986605215502));
#27114=DIRECTION('center_axis',(0.392106666069813,0.159229418444589,-0.906034411446615));
#27115=DIRECTION('ref_axis',(-0.839458305969898,-0.340893102399512,-0.423204023225896));
#27116=DIRECTION('center_axis',(-0.700067241886855,0.714076926414047,-1.13254949294063E-16));
#27117=DIRECTION('ref_axis',(4.44089209850063E-15,-4.44089209850063E-15,
-1.));
#27118=DIRECTION('center_axis',(0.,-1.58603289232165E-16,-1.));
#27119=DIRECTION('ref_axis',(-0.707106781186548,0.707106781186548,0.));
#27120=DIRECTION('',(0.,-1.58603289232165E-16,-1.));
#27121=DIRECTION('center_axis',(4.44089209850062E-15,-9.86076131526262E-30,
1.));
#27122=DIRECTION('ref_axis',(2.22044604925031E-15,1.,0.));
#27123=DIRECTION('',(0.,1.58603289232165E-16,1.));
#27124=DIRECTION('center_axis',(0.700212217679577,0.,0.71393476607618));
#27125=DIRECTION('ref_axis',(0.,1.,0.));
#27126=DIRECTION('center_axis',(1.,0.,0.));
#27127=DIRECTION('ref_axis',(0.,1.,0.));
#27128=DIRECTION('center_axis',(1.,0.,0.));
#27129=DIRECTION('ref_axis',(0.,-0.717262041981833,0.696803532663298));
#27130=DIRECTION('center_axis',(-0.70021221767957,0.713934766076186,0.));
#27131=DIRECTION('ref_axis',(0.,0.,-1.));
#27132=DIRECTION('center_axis',(0.,1.58603289232165E-16,1.));
#27133=DIRECTION('ref_axis',(0.,-1.,1.58603289232165E-16));
#27134=DIRECTION('',(-1.,0.,0.));
#27135=DIRECTION('',(0.,-1.,1.58603289232165E-16));
#27136=DIRECTION('',(1.,0.,0.));
#27137=DIRECTION('center_axis',(1.,0.,0.));
#27138=DIRECTION('ref_axis',(0.,-0.773020682523926,-0.634380819689754));
#27139=DIRECTION('',(-1.,0.,0.));
#27140=DIRECTION('center_axis',(1.,0.,0.));
#27141=DIRECTION('ref_axis',(0.,-0.980778988433322,0.195121951219513));
#27142=DIRECTION('center_axis',(1.,0.,0.));
#27143=DIRECTION('ref_axis',(0.,-0.773020682523926,-0.634380819689754));
#27144=DIRECTION('center_axis',(-0.93091161074757,0.339317183161405,0.135157027885253));
#27145=DIRECTION('ref_axis',(-0.365244538597586,-0.864829647402693,-0.344479473986434));
#27146=DIRECTION('center_axis',(0.,-0.195121951219512,-0.980778988433322));
#27147=DIRECTION('ref_axis',(0.,-0.980778988433322,0.195121951219512));
#27148=DIRECTION('center_axis',(-1.,0.,0.));
#27149=DIRECTION('ref_axis',(0.,0.,1.));
#27150=DIRECTION('center_axis',(-1.,0.,0.));
#27151=DIRECTION('ref_axis',(0.,-0.707106781186547,0.707106781186548));
#27152=DIRECTION('center_axis',(1.,0.,0.));
#27153=DIRECTION('ref_axis',(0.,0.,-1.));
#27154=DIRECTION('center_axis',(-1.,0.,0.));
#27155=DIRECTION('ref_axis',(0.,-0.717262041981833,0.696803532663298));
#27156=DIRECTION('center_axis',(2.75992815003008E-16,0.980778988433322,
0.19512195121951));
#27157=DIRECTION('ref_axis',(-0.707106781186547,-0.137972054865666,0.693515473566485));
#27158=DIRECTION('center_axis',(1.,0.,0.));
#27159=DIRECTION('ref_axis',(0.,1.,0.));
#27160=DIRECTION('center_axis',(1.,0.,0.));
#27161=DIRECTION('ref_axis',(0.,-1.,1.83697019872103E-16));
#27162=DIRECTION('',(-1.,0.,0.));
#27163=DIRECTION('center_axis',(1.,0.,0.));
#27164=DIRECTION('ref_axis',(0.,1.,0.));
#27165=DIRECTION('',(1.,0.,0.));
#27166=DIRECTION('center_axis',(1.,0.,0.));
#27167=DIRECTION('ref_axis',(0.,0.,-1.));
#27168=DIRECTION('',(-1.,0.,0.));
#27169=DIRECTION('center_axis',(-1.,0.,0.));
#27170=DIRECTION('ref_axis',(0.,-1.60812264967664E-16,-1.));
#27171=DIRECTION('',(1.,0.,0.));
#27172=DIRECTION('center_axis',(-1.,0.,0.));
#27173=DIRECTION('ref_axis',(0.,0.707106781186547,-0.707106781186548));
#27174=DIRECTION('',(-1.,0.,0.));
#27175=DIRECTION('center_axis',(1.,0.,0.));
#27176=DIRECTION('ref_axis',(0.,1.,0.));
#27177=DIRECTION('',(1.,0.,0.));
#27178=DIRECTION('center_axis',(-1.,0.,0.));
#27179=DIRECTION('ref_axis',(0.,0.707106781186548,0.707106781186547));
#27180=DIRECTION('',(-1.,0.,0.));
#27181=DIRECTION('center_axis',(-1.,0.,0.));
#27182=DIRECTION('ref_axis',(0.,6.12323399573677E-17,1.));
#27183=DIRECTION('',(1.,0.,0.));
#27184=DIRECTION('center_axis',(1.,0.,0.));
#27185=DIRECTION('ref_axis',(0.,1.,0.));
#27186=DIRECTION('center_axis',(1.,0.,0.));
#27187=DIRECTION('ref_axis',(0.,-1.,1.83697019872103E-16));
#27188=DIRECTION('center_axis',(-1.,0.,0.));
#27189=DIRECTION('ref_axis',(0.,0.773020682523925,-0.634380819689755));
#27190=DIRECTION('center_axis',(1.,0.,0.));
#27191=DIRECTION('ref_axis',(0.,0.773020682523925,-0.634380819689755));
#27192=DIRECTION('',(-1.,0.,0.));
#27193=DIRECTION('center_axis',(1.,0.,0.));
#27194=DIRECTION('ref_axis',(0.,0.,-1.));
#27195=DIRECTION('center_axis',(-0.93091161074757,-0.339317183161405,0.135157027885251));
#27196=DIRECTION('ref_axis',(-0.365244538597587,0.864829647402694,-0.344479473986432));
#27197=DIRECTION('center_axis',(0.700212217679577,0.71393476607618,0.));
#27198=DIRECTION('ref_axis',(0.,0.,-1.));
#27199=DIRECTION('center_axis',(0.,0.195121951219512,-0.980778988433322));
#27200=DIRECTION('ref_axis',(0.,0.980778988433322,0.195121951219512));
#27201=DIRECTION('center_axis',(0.392106667949502,-0.159229414617378,-0.906034411305744));
#27202=DIRECTION('ref_axis',(-0.839458309265364,0.340893093909927,-0.423204023527487));
#27203=DIRECTION('center_axis',(-0.700067241886871,-0.714076926414031,0.));
#27204=DIRECTION('ref_axis',(-0.70710678118655,0.693233845981671,0.1393801807484));
#27205=DIRECTION('center_axis',(0.,1.,0.));
#27206=DIRECTION('ref_axis',(-0.707106781186548,0.,-0.707106781186547));
#27207=DIRECTION('center_axis',(0.,0.1971133419404,-0.980380706883345));
#27208=DIRECTION('ref_axis',(0.,0.980380706883345,0.1971133419404));
#27209=DIRECTION('center_axis',(1.,0.,0.));
#27210=DIRECTION('ref_axis',(0.,0.,-1.));
#27211=DIRECTION('center_axis',(1.,3.76456815122937E-17,-3.76456815122937E-17));
#27212=DIRECTION('ref_axis',(0.,0.707106781186547,0.707106781186547));
#27213=DIRECTION('center_axis',(0.,-0.980778988433322,0.195121951219512));
#27214=DIRECTION('ref_axis',(0.,0.195121951219512,0.980778988433322));
#27215=DIRECTION('center_axis',(1.,0.,0.));
#27216=DIRECTION('ref_axis',(0.,1.,0.));
#27217=DIRECTION('center_axis',(-1.,-3.80233094921144E-17,3.80233094921144E-17));
#27218=DIRECTION('ref_axis',(0.,0.707106781186548,0.707106781186548));
#27219=DIRECTION('center_axis',(1.,0.,0.));
#27220=DIRECTION('ref_axis',(0.,0.,-1.));
#27221=DIRECTION('center_axis',(1.,0.,0.));
#27222=DIRECTION('ref_axis',(0.,0.707106781186548,0.707106781186547));
#27223=DIRECTION('center_axis',(4.56684708566872E-15,0.980380706883345,
-0.197113341940397));
#27224=DIRECTION('ref_axis',(-1.,5.55111512312578E-15,4.44089209850062E-15));
#27225=DIRECTION('center_axis',(1.,0.,0.));
#27226=DIRECTION('ref_axis',(0.,0.,-1.));
#27227=DIRECTION('center_axis',(1.,0.,0.));
#27228=DIRECTION('ref_axis',(0.,0.999895356874024,-0.0144663506721044));
#27229=DIRECTION('center_axis',(1.,0.,0.));
#27230=DIRECTION('ref_axis',(0.,0.,-1.));
#27231=DIRECTION('center_axis',(1.,0.,0.));
#27232=DIRECTION('ref_axis',(0.,0.773020682523925,0.634380819689755));
#27233=DIRECTION('',(0.,1.,0.));
#27234=DIRECTION('center_axis',(-1.,0.,0.));
#27235=DIRECTION('ref_axis',(0.,0.99994072112783,-0.0108882611263663));
#27236=DIRECTION('',(0.,-1.,0.));
#27237=DIRECTION('center_axis',(0.,0.,1.));
#27238=DIRECTION('ref_axis',(-0.772461049429072,-0.63506214429372,0.));
#27239=DIRECTION('center_axis',(-0.700067241886868,0.,0.714076926414034));
#27240=DIRECTION('ref_axis',(-0.707106781186553,0.139380180748399,-0.693233845981669));
#27241=DIRECTION('center_axis',(0.,-3.17206578464331E-16,-1.));
#27242=DIRECTION('ref_axis',(-0.707106781186548,-0.707106781186547,0.));
#27243=DIRECTION('center_axis',(0.,-0.980380706883345,-0.1971133419404));
#27244=DIRECTION('ref_axis',(0.,0.1971133419404,-0.980380706883345));
#27245=DIRECTION('center_axis',(1.,0.,0.));
#27246=DIRECTION('ref_axis',(0.,0.,-1.));
#27247=DIRECTION('center_axis',(-6.31716887673555E-15,0.980778988433321,
0.195121951219515));
#27248=DIRECTION('ref_axis',(0.,0.195121951219515,-0.980778988433321));
#27249=DIRECTION('center_axis',(1.,0.,0.));
#27250=DIRECTION('ref_axis',(0.,0.707106781186547,-0.707106781186548));
#27251=DIRECTION('center_axis',(-2.57593294002809E-15,-0.195121951219511,
-0.980778988433322));
#27252=DIRECTION('ref_axis',(-0.707106781186554,0.693515473566478,-0.137972054865664));
#27253=DIRECTION('center_axis',(0.134022231386925,-0.938793849576159,0.317339171064724));
#27254=DIRECTION('ref_axis',(-0.365244538597589,-0.344479473986443,-0.864829647402688));
#27255=DIRECTION('center_axis',(0.700212217679577,0.,-0.71393476607618));
#27256=DIRECTION('ref_axis',(0.,-1.,0.));
#27257=DIRECTION('center_axis',(-1.,0.,0.));
#27258=DIRECTION('ref_axis',(0.,-0.634380819689754,-0.773020682523925));
#27259=DIRECTION('center_axis',(-0.930911610747569,-0.339317183161406,-0.135157027885257));
#27260=DIRECTION('ref_axis',(-0.365244538597591,0.864829647402688,0.344479473986442));
#27261=DIRECTION('center_axis',(0.700212217679577,0.71393476607618,0.));
#27262=DIRECTION('ref_axis',(-0.707106781186547,0.693515473566485,-0.137972054865667));
#27263=DIRECTION('center_axis',(-1.,0.,0.));
#27264=DIRECTION('ref_axis',(0.,0.773020682523925,0.634380819689754));
#27265=DIRECTION('center_axis',(-0.392106667949504,0.159229414617379,-0.906034411305743));
#27266=DIRECTION('ref_axis',(-0.839458309265363,0.340893093909926,0.423204023527489));
#27267=DIRECTION('center_axis',(-0.700067241886868,-0.714076926414034,0.));
#27268=DIRECTION('ref_axis',(0.,0.,1.));
#27269=DIRECTION('center_axis',(0.,0.1971133419404,0.980380706883345));
#27270=DIRECTION('ref_axis',(0.,0.980380706883345,-0.1971133419404));
#27271=DIRECTION('center_axis',(0.,1.,0.));
#27272=DIRECTION('ref_axis',(-0.707106781186548,0.,0.707106781186547));
#27273=DIRECTION('center_axis',(-1.,0.,0.));
#27274=DIRECTION('ref_axis',(0.,-0.634380819689755,-0.773020682523925));
#27275=DIRECTION('center_axis',(1.,0.,0.));
#27276=DIRECTION('ref_axis',(0.,-0.634380819689755,-0.773020682523925));
#27277=DIRECTION('',(-1.,0.,0.));
#27278=DIRECTION('center_axis',(1.,0.,0.));
#27279=DIRECTION('ref_axis',(0.,0.773020682523925,0.634380819689755));
#27280=DIRECTION('',(1.,0.,0.));
#27281=DIRECTION('center_axis',(0.,0.,-1.));
#27282=DIRECTION('ref_axis',(0.,1.,0.));
#27283=DIRECTION('',(0.,1.,0.));
#27284=DIRECTION('',(-1.,0.,0.));
#27285=DIRECTION('center_axis',(0.,1.,0.));
#27286=DIRECTION('ref_axis',(-0.707106781186548,0.,0.707106781186547));
#27287=DIRECTION('',(0.,-1.,0.));
#27288=DIRECTION('center_axis',(0.,-1.,-4.44089209850063E-15));
#27289=DIRECTION('ref_axis',(-1.,0.,0.));
#27290=DIRECTION('center_axis',(1.,0.,0.));
#27291=DIRECTION('ref_axis',(0.,0.,-1.));
#27292=DIRECTION('center_axis',(1.,0.,0.));
#27293=DIRECTION('ref_axis',(0.,-0.999895356874024,-0.0144663506721044));
#27294=DIRECTION('center_axis',(1.,0.,0.));
#27295=DIRECTION('ref_axis',(0.,0.,-1.));
#27296=DIRECTION('center_axis',(-1.,0.,0.));
#27297=DIRECTION('ref_axis',(0.,-1.,-1.22464679914735E-16));
#27298=DIRECTION('',(0.,1.,0.));
#27299=DIRECTION('center_axis',(1.,0.,0.));
#27300=DIRECTION('ref_axis',(0.,-0.773020682523927,0.634380819689752));
#27301=DIRECTION('center_axis',(-0.134022231386924,-0.938793849576159,0.317339171064724));
#27302=DIRECTION('ref_axis',(-0.365244538597589,0.344479473986441,0.864829647402689));
#27303=DIRECTION('center_axis',(-1.,0.,0.));
#27304=DIRECTION('ref_axis',(0.,0.634380819689754,0.773020682523925));
#27305=DIRECTION('center_axis',(0.,0.,1.));
#27306=DIRECTION('ref_axis',(1.,0.,0.));
#27307=DIRECTION('center_axis',(-1.,0.,0.));
#27308=DIRECTION('ref_axis',(0.,0.777986605215495,-0.628280862437548));
#27309=DIRECTION('center_axis',(0.,0.977588190579301,0.210526315789473));
#27310=DIRECTION('ref_axis',(0.,-0.210526315789474,0.977588190579301));
#27311=DIRECTION('center_axis',(1.,0.,0.));
#27312=DIRECTION('ref_axis',(0.,0.777986605215496,-0.628280862437547));
#27313=DIRECTION('',(1.,0.,0.));
#27314=DIRECTION('',(-1.,0.,0.));
#27315=DIRECTION('center_axis',(0.,-1.,1.58603289232165E-16));
#27316=DIRECTION('ref_axis',(0.,-1.58603289232165E-16,-1.));
#27317=DIRECTION('',(-1.,0.,0.));
#27318=DIRECTION('',(0.,-1.58603289232165E-16,-1.));
#27319=DIRECTION('center_axis',(-1.,0.,0.));
#27320=DIRECTION('ref_axis',(0.,0.634380819689755,0.773020682523925));
#27321=DIRECTION('center_axis',(-1.,0.,0.));
#27322=DIRECTION('ref_axis',(0.,0.634380819689755,0.773020682523925));
#27323=DIRECTION('center_axis',(0.,0.,1.));
#27324=DIRECTION('ref_axis',(-0.772461049429072,-0.63506214429372,0.));
#27325=DIRECTION('center_axis',(-0.700067241886871,0.,-0.714076926414031));
#27326=DIRECTION('ref_axis',(0.,-1.,0.));
#27327=DIRECTION('center_axis',(0.,1.58603289232165E-16,1.));
#27328=DIRECTION('ref_axis',(-0.707106781186548,-0.707106781186547,0.));
#27329=DIRECTION('center_axis',(-0.700212217664035,0.,-0.713934766091423));
#27330=DIRECTION('ref_axis',(0.,-1.,0.));
#27331=DIRECTION('center_axis',(1.,0.,0.));
#27332=DIRECTION('ref_axis',(0.,-0.634380819689754,0.773020682523926));
#27333=DIRECTION('center_axis',(1.,0.,0.));
#27334=DIRECTION('ref_axis',(0.,0.195121951219513,0.980778988433322));
#27335=DIRECTION('',(1.,0.,0.));
#27336=DIRECTION('center_axis',(-1.,0.,0.));
#27337=DIRECTION('ref_axis',(0.,-0.634380819689754,0.773020682523926));
#27338=DIRECTION('center_axis',(1.,0.,0.));
#27339=DIRECTION('ref_axis',(0.,-1.22464679914735E-16,1.));
#27340=DIRECTION('center_axis',(1.,0.,0.));
#27341=DIRECTION('ref_axis',(0.,6.12323399573676E-17,1.));
#27342=DIRECTION('center_axis',(0.134022265816183,-0.938793848267554,-0.317339160395456));
#27343=DIRECTION('ref_axis',(-0.365244628135662,-0.344479477552722,0.864829608167439));
#27344=DIRECTION('center_axis',(0.,1.,-1.58603289232165E-16));
#27345=DIRECTION('ref_axis',(0.,1.58603289232165E-16,1.));
#27346=DIRECTION('',(0.,1.58603289232165E-16,1.));
#27347=DIRECTION('',(-1.,0.,0.));
#27348=DIRECTION('',(0.,1.58603289232165E-16,1.));
#27349=DIRECTION('center_axis',(0.,1.58603289232165E-16,1.));
#27350=DIRECTION('ref_axis',(-0.707106781186548,-0.707106781186548,0.));
#27351=DIRECTION('',(0.,-1.58603289232165E-16,-1.));
#27352=DIRECTION('center_axis',(0.,0.,1.));
#27353=DIRECTION('ref_axis',(-1.,0.,0.));
#27354=DIRECTION('center_axis',(-1.,0.,0.));
#27355=DIRECTION('ref_axis',(0.,0.,1.));
#27356=DIRECTION('',(0.,1.,0.));
#27357=DIRECTION('center_axis',(-1.,0.,0.));
#27358=DIRECTION('ref_axis',(0.,0.714764027971838,0.699365701416271));
#27359=DIRECTION('center_axis',(0.,-1.,0.));
#27360=DIRECTION('ref_axis',(-0.707106781186548,0.,-0.707106781186547));
#27361=DIRECTION('',(0.,-1.,0.));
#27362=DIRECTION('center_axis',(0.,1.,0.));
#27363=DIRECTION('ref_axis',(2.22044604925031E-15,0.,-1.));
#27364=DIRECTION('center_axis',(0.336615931322928,-0.848909755674504,0.407482443180381));
#27365=DIRECTION('ref_axis',(-0.540654873563249,-0.528537819574587,-0.654476952208134));
#27366=DIRECTION('center_axis',(-1.,0.,0.));
#27367=DIRECTION('ref_axis',(0.,-0.628280862437545,-0.777986605215498));
#27368=DIRECTION('center_axis',(0.,0.210526315789474,-0.977588190579301));
#27369=DIRECTION('ref_axis',(0.,0.977588190579301,0.210526315789474));
#27370=DIRECTION('center_axis',(1.,0.,0.));
#27371=DIRECTION('ref_axis',(0.,0.,-1.));
#27372=DIRECTION('center_axis',(1.,0.,0.));
#27373=DIRECTION('ref_axis',(0.,-1.60812264967664E-16,-1.));
#27374=DIRECTION('center_axis',(1.,0.,0.));
#27375=DIRECTION('ref_axis',(0.,0.,-1.));
#27376=DIRECTION('center_axis',(1.,0.,0.));
#27377=DIRECTION('ref_axis',(0.,0.634380819689754,-0.773020682523926));
#27378=DIRECTION('',(0.,-3.17206578464331E-16,-1.));
#27379=DIRECTION('center_axis',(-1.,0.,0.));
#27380=DIRECTION('ref_axis',(0.,-1.60812264967664E-16,-1.));
#27381=DIRECTION('',(0.,3.17206578464331E-16,1.));
#27382=DIRECTION('center_axis',(-1.,0.,0.));
#27383=DIRECTION('ref_axis',(0.,-1.22464679914735E-16,-1.));
#27384=DIRECTION('center_axis',(1.,0.,0.));
#27385=DIRECTION('ref_axis',(0.,-1.60812264967664E-16,-1.));
#27386=DIRECTION('center_axis',(1.,0.,0.));
#27387=DIRECTION('ref_axis',(0.,0.,-1.));
#27388=DIRECTION('center_axis',(1.,0.,0.));
#27389=DIRECTION('ref_axis',(0.,0.714764027971838,0.699365701416271));
#27390=DIRECTION('center_axis',(0.,0.9775881905793,-0.210526315789475));
#27391=DIRECTION('ref_axis',(0.,-0.210526315789475,-0.9775881905793));
#27392=DIRECTION('center_axis',(1.,0.,0.));
#27393=DIRECTION('ref_axis',(0.,-0.628280862437546,-0.777986605215497));
#27394=DIRECTION('',(1.,0.,0.));
#27395=DIRECTION('',(-1.,0.,0.));
#27396=DIRECTION('center_axis',(-1.,0.,0.));
#27397=DIRECTION('ref_axis',(0.,0.,1.));
#27398=DIRECTION('center_axis',(1.,0.,0.));
#27399=DIRECTION('ref_axis',(0.,0.99994072112783,-0.0108882611263663));
#27400=DIRECTION('center_axis',(0.,0.,1.));
#27401=DIRECTION('ref_axis',(-0.70710678118655,0.707106781186545,0.));
#27402=DIRECTION('center_axis',(-1.,0.,0.));
#27403=DIRECTION('ref_axis',(0.,-0.777986605215498,-0.628280862437545));
#27404=DIRECTION('center_axis',(-1.,0.,0.));
#27405=DIRECTION('ref_axis',(0.,-0.777986605215497,-0.628280862437546));
#27406=DIRECTION('',(1.,0.,0.));
#27407=DIRECTION('center_axis',(1.,0.,0.));
#27408=DIRECTION('ref_axis',(0.,1.,0.));
#27409=DIRECTION('',(-1.,0.,0.));
#27410=DIRECTION('',(-1.,0.,0.));
#27411=DIRECTION('center_axis',(-1.,0.,0.));
#27412=DIRECTION('ref_axis',(0.,0.715194520129579,0.698925459814293));
#27413=DIRECTION('',(-1.,0.,0.));
#27414=DIRECTION('',(-1.,0.,0.));
#27415=DIRECTION('center_axis',(-1.,0.,0.));
#27416=DIRECTION('ref_axis',(0.,-0.698925459814292,0.71519452012958));
#27417=DIRECTION('',(-1.,0.,0.));
#27418=DIRECTION('',(-1.,0.,0.));
#27419=DIRECTION('center_axis',(1.,0.,0.));
#27420=DIRECTION('ref_axis',(0.,-1.,-1.22464679914735E-16));
#27421=DIRECTION('',(1.,0.,0.));
#27422=DIRECTION('center_axis',(1.,0.,0.));
#27423=DIRECTION('ref_axis',(0.,-0.707106781186547,0.707106781186548));
#27424=DIRECTION('center_axis',(1.,0.,0.));
#27425=DIRECTION('ref_axis',(0.,6.12323399573677E-17,1.));
#27426=DIRECTION('',(-1.,0.,0.));
#27427=DIRECTION('center_axis',(1.,0.,0.));
#27428=DIRECTION('ref_axis',(0.,0.707106781186547,-0.707106781186548));
#27429=DIRECTION('',(1.,0.,0.));
#27430=DIRECTION('',(-1.,0.,0.));
#27431=DIRECTION('center_axis',(1.,0.,0.));
#27432=DIRECTION('ref_axis',(0.,-0.716797558008402,-0.697281335497511));
#27433=DIRECTION('',(-1.,0.,0.));
#27434=DIRECTION('center_axis',(1.,0.,0.));
#27435=DIRECTION('ref_axis',(0.,-1.,-1.22464679914735E-16));
#27436=DIRECTION('',(1.,0.,0.));
#27437=DIRECTION('center_axis',(-1.,0.,0.));
#27438=DIRECTION('ref_axis',(0.,-0.707106781186547,-0.707106781186548));
#27439=DIRECTION('',(-1.,0.,0.));
#27440=DIRECTION('',(-1.,0.,0.));
#27441=DIRECTION('center_axis',(-1.,0.,0.));
#27442=DIRECTION('ref_axis',(0.,0.698925459814293,-0.71519452012958));
#27443=DIRECTION('center_axis',(1.,0.,0.));
#27444=DIRECTION('ref_axis',(0.,-0.996859054590094,-0.0791961191078487));
#27445=DIRECTION('',(1.,0.,0.));
#27446=DIRECTION('center_axis',(1.,0.,0.));
#27447=DIRECTION('ref_axis',(0.,0.,-1.));
#27448=DIRECTION('center_axis',(1.,0.,0.));
#27449=DIRECTION('ref_axis',(0.,0.698925459814293,-0.71519452012958));
#27450=DIRECTION('center_axis',(1.,0.,0.));
#27451=DIRECTION('ref_axis',(0.,0.,-1.));
#27452=DIRECTION('',(0.,0.707106781186548,-0.707106781186548));
#27453=DIRECTION('',(0.,0.707106781186548,0.707106781186548));
#27454=DIRECTION('',(0.,-0.707106781186548,0.707106781186548));
#27455=DIRECTION('center_axis',(1.,0.,0.));
#27456=DIRECTION('ref_axis',(0.,0.996859054590094,0.0791961191078482));
#27457=DIRECTION('',(1.,0.,0.));
#27458=DIRECTION('center_axis',(1.,0.,0.));
#27459=DIRECTION('ref_axis',(0.,0.,-1.));
#27460=DIRECTION('center_axis',(1.,0.,0.));
#27461=DIRECTION('ref_axis',(0.,-0.698925459814292,0.71519452012958));
#27462=DIRECTION('center_axis',(1.,0.,0.));
#27463=DIRECTION('ref_axis',(0.,0.,-1.));
#27464=DIRECTION('',(0.,-0.707106781186548,0.707106781186548));
#27465=DIRECTION('',(0.,-0.707106781186548,-0.707106781186547));
#27466=DIRECTION('',(0.,0.707106781186548,-0.707106781186547));
#27467=DIRECTION('center_axis',(-1.,0.,0.));
#27468=DIRECTION('ref_axis',(0.,0.62828086243754,-0.777986605215502));
#27469=DIRECTION('center_axis',(1.,0.,0.));
#27470=DIRECTION('ref_axis',(0.,0.,-1.));
#27471=DIRECTION('center_axis',(-4.34136367113112E-15,-0.977588190579299,
0.210526315789481));
#27472=DIRECTION('ref_axis',(0.,0.210526315789481,0.977588190579299));
#27473=DIRECTION('center_axis',(-1.,0.,0.));
#27474=DIRECTION('ref_axis',(0.,-0.716797558008402,-0.697281335497511));
#27475=DIRECTION('center_axis',(0.,0.,1.));
#27476=DIRECTION('ref_axis',(-0.707106781186549,0.707106781186546,0.));
#27477=DIRECTION('center_axis',(-1.,0.,0.));
#27478=DIRECTION('ref_axis',(0.,0.777986605215498,0.628280862437544));
#27479=DIRECTION('center_axis',(0.,3.17206578464331E-16,1.));
#27480=DIRECTION('ref_axis',(-0.707106781186548,0.707106781186547,0.));
#27481=DIRECTION('center_axis',(1.,0.,0.));
#27482=DIRECTION('ref_axis',(0.,0.628280862437546,0.777986605215497));
#27483=DIRECTION('',(1.,0.,0.));
#27484=DIRECTION('center_axis',(-1.,0.,0.));
#27485=DIRECTION('ref_axis',(0.,0.,1.));
#27486=DIRECTION('center_axis',(1.,0.,0.));
#27487=DIRECTION('ref_axis',(0.,0.,-1.));
#27488=DIRECTION('center_axis',(-1.,0.,0.));
#27489=DIRECTION('ref_axis',(0.,0.,1.));
#27490=DIRECTION('center_axis',(-1.,0.,0.));
#27491=DIRECTION('ref_axis',(0.,6.12323399573677E-17,1.));
#27492=DIRECTION('center_axis',(1.,0.,0.));
#27493=DIRECTION('ref_axis',(0.,0.,-1.));
#27494=DIRECTION('center_axis',(-1.,0.,0.));
#27495=DIRECTION('ref_axis',(0.,0.777986605215499,0.628280862437544));
#27496=DIRECTION('',(-1.,0.,0.));
#27497=DIRECTION('center_axis',(0.,-3.17206578464331E-16,-1.));
#27498=DIRECTION('ref_axis',(-0.707106781186548,0.707106781186548,0.));
#27499=DIRECTION('',(0.,-3.17206578464331E-16,-1.));
#27500=DIRECTION('center_axis',(0.,0.,1.));
#27501=DIRECTION('ref_axis',(2.22044604925031E-15,1.,0.));
#27502=DIRECTION('',(0.,3.17206578464331E-16,1.));
#27503=DIRECTION('center_axis',(0.472949929361147,-0.380667016315068,-0.794613734469189));
#27504=DIRECTION('ref_axis',(-0.619013384421907,0.498230285022508,-0.607115320999995));
#27505=DIRECTION('center_axis',(-1.,0.,0.));
#27506=DIRECTION('ref_axis',(0.,0.634380819689754,-0.773020682523926));
#27507=DIRECTION('center_axis',(1.,0.,0.));
#27508=DIRECTION('ref_axis',(0.,0.634380819689754,-0.773020682523926));
#27509=DIRECTION('',(1.,0.,0.));
#27510=DIRECTION('center_axis',(0.,-1.,3.17206578464331E-16));
#27511=DIRECTION('ref_axis',(0.,-3.17206578464331E-16,-1.));
#27512=DIRECTION('center_axis',(1.,0.,0.));
#27513=DIRECTION('ref_axis',(0.,0.,-1.));
#27514=DIRECTION('center_axis',(1.,0.,0.));
#27515=DIRECTION('ref_axis',(0.,0.707106781186547,-0.707106781186548));
#27516=DIRECTION('center_axis',(-1.,0.,0.));
#27517=DIRECTION('ref_axis',(0.,0.707106781186547,-0.707106781186548));
#27518=DIRECTION('center_axis',(-1.,0.,0.));
#27519=DIRECTION('ref_axis',(0.,0.,1.));
#27520=DIRECTION('',(0.,-3.17206578464331E-16,-1.));
#27521=DIRECTION('center_axis',(-1.,0.,0.));
#27522=DIRECTION('ref_axis',(0.,0.707106781186547,-0.707106781186548));
#27523=DIRECTION('center_axis',(0.,3.17206578464331E-16,1.));
#27524=DIRECTION('ref_axis',(-0.707106781186548,-0.707106781186548,0.));
#27525=DIRECTION('',(0.,3.17206578464331E-16,1.));
#27526=DIRECTION('center_axis',(-4.44089209850062E-15,0.,1.));
#27527=DIRECTION('ref_axis',(0.,-1.,0.));
#27528=DIRECTION('center_axis',(0.,0.,1.));
#27529=DIRECTION('ref_axis',(1.,0.,0.));
#27530=DIRECTION('center_axis',(-1.,0.,0.));
#27531=DIRECTION('ref_axis',(0.,-0.210526315789473,0.977588190579301));
#27532=DIRECTION('center_axis',(0.,-0.977588190579299,-0.210526315789481));
#27533=DIRECTION('ref_axis',(-1.,0.,0.));
#27534=DIRECTION('center_axis',(0.336615931322922,-0.848909755674508,-0.407482443180376));
#27535=DIRECTION('ref_axis',(-0.540654873563252,-0.528537819574574,0.654476952208142));
#27536=DIRECTION('center_axis',(6.51204550669669E-15,0.210526315789473,
0.977588190579301));
#27537=DIRECTION('ref_axis',(0.,-0.977588190579301,0.210526315789473));
#27538=DIRECTION('center_axis',(-1.,0.,0.));
#27539=DIRECTION('ref_axis',(0.,0.,1.));
#27540=DIRECTION('center_axis',(-1.,0.,0.));
#27541=DIRECTION('ref_axis',(0.,-0.628280862437546,0.777986605215497));
#27542=DIRECTION('center_axis',(1.,0.,0.));
#27543=DIRECTION('ref_axis',(0.,0.,-1.));
#27544=DIRECTION('center_axis',(1.,0.,0.));
#27545=DIRECTION('ref_axis',(0.,-0.777986605215497,0.628280862437546));
#27546=DIRECTION('',(1.,0.,0.));
#27547=DIRECTION('center_axis',(0.,1.,-3.17206578464331E-16));
#27548=DIRECTION('ref_axis',(0.,3.17206578464331E-16,1.));
#27549=DIRECTION('center_axis',(-1.,0.,0.));
#27550=DIRECTION('ref_axis',(0.,0.,1.));
#27551=DIRECTION('center_axis',(1.,0.,0.));
#27552=DIRECTION('ref_axis',(0.,0.,-1.));
#27553=DIRECTION('center_axis',(1.,0.,0.));
#27554=DIRECTION('ref_axis',(0.,-0.773020682523927,0.634380819689752));
#27555=DIRECTION('',(0.,1.,0.));
#27556=DIRECTION('center_axis',(-1.,0.,0.));
#27557=DIRECTION('ref_axis',(0.,-0.773020682523927,0.634380819689752));
#27558=DIRECTION('',(-1.,0.,0.));
#27559=DIRECTION('center_axis',(0.,0.,-1.));
#27560=DIRECTION('ref_axis',(0.,1.,0.));
#27561=DIRECTION('center_axis',(1.,0.,0.));
#27562=DIRECTION('ref_axis',(0.,0.0791961191078487,-0.996859054590094));
#27563=DIRECTION('',(1.,0.,0.));
#27564=DIRECTION('center_axis',(0.,-0.707106781186548,0.707106781186548));
#27565=DIRECTION('ref_axis',(0.,-0.707106781186548,-0.707106781186548));
#27566=DIRECTION('',(0.,-0.707106781186548,-0.707106781186548));
#27567=DIRECTION('',(1.,0.,0.));
#27568=DIRECTION('',(0.,0.707106781186548,0.707106781186548));
#27569=DIRECTION('',(1.,0.,0.));
#27570=DIRECTION('center_axis',(1.,0.,0.));
#27571=DIRECTION('ref_axis',(0.,0.,-1.));
#27572=DIRECTION('center_axis',(1.,0.,0.));
#27573=DIRECTION('ref_axis',(0.,0.71519452012958,0.698925459814293));
#27574=DIRECTION('center_axis',(1.,0.,0.));
#27575=DIRECTION('ref_axis',(0.,0.,-1.));
#27576=DIRECTION('',(0.,0.707106781186548,0.707106781186548));
#27577=DIRECTION('',(0.,-0.707106781186548,0.707106781186548));
#27578=DIRECTION('center_axis',(1.,0.,0.));
#27579=DIRECTION('ref_axis',(0.,0.,-1.));
#27580=DIRECTION('center_axis',(-1.,0.,0.));
#27581=DIRECTION('ref_axis',(0.,-1.,3.06161699786838E-17));
#27582=DIRECTION('center_axis',(-1.,0.,0.));
#27583=DIRECTION('ref_axis',(0.,-1.,3.06161699786838E-17));
#27584=DIRECTION('center_axis',(0.,-1.,-1.22464679914735E-16));
#27585=DIRECTION('ref_axis',(0.,-1.22464679914735E-16,1.));
#27586=DIRECTION('center_axis',(-1.,0.,0.));
#27587=DIRECTION('ref_axis',(0.,1.,0.));
#27588=DIRECTION('center_axis',(1.,0.,0.));
#27589=DIRECTION('ref_axis',(0.,-1.,3.06161699786838E-17));
#27590=DIRECTION('',(-0.707106781186548,-0.707106781186548,-8.65956056235493E-17));
#27591=DIRECTION('center_axis',(1.,0.,0.));
#27592=DIRECTION('ref_axis',(0.,-1.,3.06161699786838E-17));
#27593=DIRECTION('center_axis',(1.,0.,0.));
#27594=DIRECTION('ref_axis',(0.,-1.,3.06161699786838E-17));
#27595=DIRECTION('center_axis',(1.,0.,0.));
#27596=DIRECTION('ref_axis',(0.,-1.,3.06161699786838E-17));
#27597=DIRECTION('center_axis',(-1.,0.,0.));
#27598=DIRECTION('ref_axis',(0.,-0.0791961191078482,-0.996859054590094));
#27599=DIRECTION('',(-1.,0.,0.));
#27600=DIRECTION('center_axis',(0.,0.707106781186548,0.707106781186548));
#27601=DIRECTION('ref_axis',(0.,-0.707106781186548,0.707106781186548));
#27602=DIRECTION('',(-1.,0.,0.));
#27603=DIRECTION('',(0.,-0.707106781186548,0.707106781186548));
#27604=DIRECTION('',(1.,0.,0.));
#27605=DIRECTION('center_axis',(-1.,0.,0.));
#27606=DIRECTION('ref_axis',(0.,-0.996859054590094,0.0791961191078482));
#27607=DIRECTION('',(-1.,0.,0.));
#27608=DIRECTION('center_axis',(0.,0.707106781186548,-0.707106781186548));
#27609=DIRECTION('ref_axis',(0.,0.707106781186548,0.707106781186548));
#27610=DIRECTION('',(-1.,0.,0.));
#27611=DIRECTION('',(0.,0.707106781186547,0.707106781186547));
#27612=DIRECTION('',(1.,0.,0.));
#27613=DIRECTION('center_axis',(-1.,0.,0.));
#27614=DIRECTION('ref_axis',(0.,0.0791961191078487,0.996859054590094));
#27615=DIRECTION('',(-1.,0.,0.));
#27616=DIRECTION('center_axis',(0.,-0.707106781186548,-0.707106781186548));
#27617=DIRECTION('ref_axis',(0.,0.707106781186548,-0.707106781186548));
#27618=DIRECTION('',(-1.,0.,0.));
#27619=DIRECTION('',(0.,0.707106781186548,-0.707106781186548));
#27620=DIRECTION('',(1.,0.,0.));
#27621=DIRECTION('center_axis',(0.,-0.707106781186547,-0.707106781186548));
#27622=DIRECTION('ref_axis',(0.707106781186544,-0.500000000000003,0.500000000000002));
#27623=DIRECTION('',(0.,0.707106781186547,0.707106781186548));
#27624=DIRECTION('center_axis',(0.,-0.707106781186548,-0.707106781186548));
#27625=DIRECTION('ref_axis',(1.,0.,0.));
#27626=DIRECTION('',(0.,-0.707106781186547,-0.707106781186548));
#27627=DIRECTION('center_axis',(0.,-1.,-6.28036983473513E-15));
#27628=DIRECTION('ref_axis',(-1.96261557335473E-16,-6.31439345255561E-15,
1.));
#27629=DIRECTION('center_axis',(1.,0.,0.));
#27630=DIRECTION('ref_axis',(0.,0.,-1.));
#27631=DIRECTION('center_axis',(-1.,0.,0.));
#27632=DIRECTION('ref_axis',(0.,0.0115039628724714,-0.999933827229697));
#27633=DIRECTION('center_axis',(0.,0.809885237104279,-0.586588358834836));
#27634=DIRECTION('ref_axis',(0.,0.586588358834836,0.809885237104279));
#27635=DIRECTION('center_axis',(1.,0.,0.));
#27636=DIRECTION('ref_axis',(0.,0.0115039628724714,-0.999933827229697));
#27637=DIRECTION('center_axis',(-0.0364266962331357,-0.997807365125386,
-0.055259007438373));
#27638=DIRECTION('ref_axis',(0.549169647365281,-0.0661850595039047,0.833085971740707));
#27639=DIRECTION('center_axis',(1.,0.,0.));
#27640=DIRECTION('ref_axis',(0.,-0.0791961191078493,0.996859054590094));
#27641=DIRECTION('center_axis',(1.,0.,0.));
#27642=DIRECTION('ref_axis',(0.,-0.0791961191078487,0.996859054590094));
#27643=DIRECTION('',(-1.,0.,0.));
#27644=DIRECTION('',(1.,0.,0.));
#27645=DIRECTION('center_axis',(1.,0.,0.));
#27646=DIRECTION('ref_axis',(0.,1.,0.));
#27647=DIRECTION('center_axis',(1.,0.,0.));
#27648=DIRECTION('ref_axis',(0.,0.,-1.));
#27649=DIRECTION('center_axis',(-1.,0.,0.));
#27650=DIRECTION('ref_axis',(0.,-1.,1.83697019872103E-16));
#27651=DIRECTION('center_axis',(0.,0.707106781186548,-0.707106781186548));
#27652=DIRECTION('ref_axis',(0.,0.707106781186548,0.707106781186548));
#27653=DIRECTION('',(1.,0.,0.));
#27654=DIRECTION('center_axis',(1.,0.,0.));
#27655=DIRECTION('ref_axis',(0.,0.,-1.));
#27656=DIRECTION('center_axis',(-1.,0.,0.));
#27657=DIRECTION('ref_axis',(0.,-1.,1.83697019872103E-16));
#27658=DIRECTION('center_axis',(1.,0.,0.));
#27659=DIRECTION('ref_axis',(0.,0.,-1.));
#27660=DIRECTION('',(0.,0.707106781186548,-0.707106781186548));
#27661=DIRECTION('center_axis',(1.,0.,0.));
#27662=DIRECTION('ref_axis',(0.,1.,-2.83276944882399E-16));
#27663=DIRECTION('center_axis',(1.,0.,0.));
#27664=DIRECTION('ref_axis',(0.,0.,-1.));
#27665=DIRECTION('center_axis',(-1.,0.,0.));
#27666=DIRECTION('ref_axis',(0.,1.,-2.83276944882399E-16));
#27667=DIRECTION('center_axis',(0.,0.707106781186548,0.707106781186548));
#27668=DIRECTION('ref_axis',(0.,-0.707106781186548,0.707106781186548));
#27669=DIRECTION('center_axis',(1.,0.,0.));
#27670=DIRECTION('ref_axis',(0.,1.22464679914735E-16,1.));
#27671=DIRECTION('center_axis',(-1.,0.,0.));
#27672=DIRECTION('ref_axis',(0.,-1.,1.83697019872103E-16));
#27673=DIRECTION('center_axis',(1.,0.,0.));
#27674=DIRECTION('ref_axis',(0.,0.,-1.));
#27675=DIRECTION('center_axis',(1.,0.,0.));
#27676=DIRECTION('ref_axis',(0.,1.22464679914735E-16,1.));
#27677=DIRECTION('center_axis',(1.,0.,0.));
#27678=DIRECTION('ref_axis',(0.,-1.22464679914735E-16,1.));
#27679=DIRECTION('center_axis',(-1.,0.,0.));
#27680=DIRECTION('ref_axis',(0.,1.22464679914735E-16,1.));
#27681=DIRECTION('center_axis',(0.,-0.707106781186547,0.707106781186548));
#27682=DIRECTION('ref_axis',(0.,-0.707106781186548,-0.707106781186547));
#27683=DIRECTION('',(1.,0.,0.));
#27684=DIRECTION('center_axis',(1.,0.,0.));
#27685=DIRECTION('ref_axis',(0.,0.,-1.));
#27686=DIRECTION('',(0.,-0.707106781186548,0.707106781186547));
#27687=DIRECTION('center_axis',(-1.,0.,0.));
#27688=DIRECTION('ref_axis',(0.,-1.,1.83697019872103E-16));
#27689=DIRECTION('',(0.,-0.707106781186548,-0.707106781186548));
#27690=DIRECTION('center_axis',(1.,0.,0.));
#27691=DIRECTION('ref_axis',(0.,-0.999933827229697,0.0115039628724727));
#27692=DIRECTION('center_axis',(1.,0.,0.));
#27693=DIRECTION('ref_axis',(0.,0.,-1.));
#27694=DIRECTION('center_axis',(0.,-0.586588358834838,0.809885237104277));
#27695=DIRECTION('ref_axis',(1.,0.,0.));
#27696=DIRECTION('center_axis',(-1.,0.,0.));
#27697=DIRECTION('ref_axis',(0.,-0.999933827229697,0.0115039628724727));
#27698=DIRECTION('center_axis',(0.,0.707106781186548,0.707106781186548));
#27699=DIRECTION('ref_axis',(0.707106781186547,0.500000000000001,-0.5));
#27700=DIRECTION('center_axis',(0.,3.14018491736755E-15,-1.));
#27701=DIRECTION('ref_axis',(-1.47196168001603E-16,1.,3.12250225675824E-15));
#27702=DIRECTION('',(0.,0.707106781186548,0.707106781186548));
#27703=DIRECTION('center_axis',(0.,-0.707106781186543,-0.707106781186552));
#27704=DIRECTION('ref_axis',(0.,0.707106781186552,-0.707106781186543));
#27705=DIRECTION('center_axis',(0.,0.,1.));
#27706=DIRECTION('ref_axis',(1.,0.,0.));
#27707=DIRECTION('center_axis',(1.,0.,0.));
#27708=DIRECTION('ref_axis',(0.,0.996859054590094,-0.0791961191078493));
#27709=DIRECTION('center_axis',(1.,0.,0.));
#27710=DIRECTION('ref_axis',(0.,-0.999933827229697,0.0115039628724726));
#27711=DIRECTION('',(1.,0.,0.));
#27712=DIRECTION('',(1.,0.,0.));
#27713=DIRECTION('center_axis',(-1.,0.,0.));
#27714=DIRECTION('ref_axis',(0.,0.996859054590094,-0.0791961191078487));
#27715=DIRECTION('',(-1.,0.,0.));
#27716=DIRECTION('center_axis',(0.,-0.707106781186548,0.707106781186548));
#27717=DIRECTION('ref_axis',(0.,-0.707106781186548,-0.707106781186548));
#27718=DIRECTION('',(1.,0.,0.));
#27719=DIRECTION('',(0.,-0.707106781186548,-0.707106781186548));
#27720=DIRECTION('',(-1.,0.,0.));
#27721=DIRECTION('center_axis',(0.,-0.707106781186548,0.707106781186548));
#27722=DIRECTION('ref_axis',(-0.707106781186547,-0.5,-0.5));
#27723=DIRECTION('',(1.,0.,0.));
#27724=DIRECTION('center_axis',(0.,-0.707106781186548,0.707106781186548));
#27725=DIRECTION('ref_axis',(0.707106781186547,-0.5,-0.5));
#27726=DIRECTION('center_axis',(1.,0.,0.));
#27727=DIRECTION('ref_axis',(0.,0.,-1.));
#27728=DIRECTION('center_axis',(0.,-0.707106781186547,0.707106781186548));
#27729=DIRECTION('ref_axis',(0.707106781186547,0.5,0.5));
#27730=DIRECTION('',(0.,-0.707106781186547,0.707106781186548));
#27731=DIRECTION('center_axis',(0.,0.707106781186548,-0.707106781186547));
#27732=DIRECTION('ref_axis',(0.,0.707106781186547,0.707106781186548));
#27733=DIRECTION('center_axis',(0.,0.707106781186548,-0.707106781186547));
#27734=DIRECTION('ref_axis',(0.707106781186547,-0.5,-0.5));
#27735=DIRECTION('',(1.,0.,0.));
#27736=DIRECTION('center_axis',(0.,0.707106781186548,-0.707106781186547));
#27737=DIRECTION('ref_axis',(-0.707106781186547,-0.5,-0.5));
#27738=DIRECTION('',(1.,0.,0.));
#27739=DIRECTION('',(0.,0.707106781186547,0.707106781186548));
#27740=DIRECTION('',(1.,0.,0.));
#27741=DIRECTION('center_axis',(0.,-0.707106781186548,-0.707106781186547));
#27742=DIRECTION('ref_axis',(0.,0.707106781186547,-0.707106781186548));
#27743=DIRECTION('',(0.,0.707106781186547,-0.707106781186548));
#27744=DIRECTION('center_axis',(0.,-0.707106781186548,0.707106781186548));
#27745=DIRECTION('ref_axis',(-0.707106781186547,-0.5,-0.5));
#27746=DIRECTION('',(0.,-0.707106781186548,0.707106781186548));
#27747=DIRECTION('center_axis',(0.,0.707106781186548,0.707106781186548));
#27748=DIRECTION('ref_axis',(0.,-0.707106781186548,0.707106781186548));
#27749=DIRECTION('',(0.,0.707106781186548,-0.707106781186548));
#27750=DIRECTION('center_axis',(0.,0.707106781186548,-0.707106781186548));
#27751=DIRECTION('ref_axis',(0.707106781186547,-0.5,-0.5));
#27752=DIRECTION('center_axis',(-1.,0.,0.));
#27753=DIRECTION('ref_axis',(0.,0.996859054590094,-0.0791961191078487));
#27754=DIRECTION('center_axis',(1.,0.,0.));
#27755=DIRECTION('ref_axis',(0.,-0.0791961191078487,0.996859054590094));
#27756=DIRECTION('center_axis',(1.,0.,0.));
#27757=DIRECTION('ref_axis',(0.,0.,-1.));
#27758=DIRECTION('center_axis',(1.,0.,0.));
#27759=DIRECTION('ref_axis',(0.,-0.707106781186548,-0.707106781186548));
#27760=DIRECTION('center_axis',(1.,0.,0.));
#27761=DIRECTION('ref_axis',(0.,0.,-1.));
#27762=DIRECTION('center_axis',(0.,-0.707106781186547,-0.707106781186548));
#27763=DIRECTION('ref_axis',(0.,0.707106781186548,-0.707106781186547));
#27764=DIRECTION('center_axis',(0.,0.707106781186548,0.707106781186548));
#27765=DIRECTION('ref_axis',(0.,-0.707106781186548,0.707106781186548));
#27766=DIRECTION('',(1.,0.,0.));
#27767=DIRECTION('center_axis',(1.,0.,0.));
#27768=DIRECTION('ref_axis',(0.,1.,0.));
#27769=DIRECTION('center_axis',(1.,0.,0.));
#27770=DIRECTION('ref_axis',(0.,1.,0.));
#27771=DIRECTION('center_axis',(0.,0.,1.));
#27772=DIRECTION('ref_axis',(0.,-1.,0.));
#27773=DIRECTION('center_axis',(1.,0.,0.));
#27774=DIRECTION('ref_axis',(0.,1.,0.));
#27775=DIRECTION('center_axis',(1.,0.,0.));
#27776=DIRECTION('ref_axis',(0.,1.,0.));
#63527=CARTESIAN_POINT('',(0.,0.,0.));
#63528=CARTESIAN_POINT('Origin',(18.5,0.,0.));
#63529=CARTESIAN_POINT('',(18.,-1.16341445918999E-15,9.5));
#63530=CARTESIAN_POINT('Origin',(18.,0.,0.));
#63531=CARTESIAN_POINT('',(18.5,-1.10218211923262E-15,9.));
#63532=CARTESIAN_POINT('Origin',(18.5,-1.16341445918999E-15,9.5));
#63533=CARTESIAN_POINT('',(18.5,-9.,-1.10218211923262E-15));
#63534=CARTESIAN_POINT('Origin',(18.5,0.,0.));
#63535=CARTESIAN_POINT('Origin',(18.5,0.,0.));
#63536=CARTESIAN_POINT('Origin',(19.5,0.,0.));
#63537=CARTESIAN_POINT('',(20.5,-1.10218211923262E-15,9.));
#63538=CARTESIAN_POINT('',(20.5,-9.,-1.10218211923262E-15));
#63539=CARTESIAN_POINT('Origin',(20.5,0.,0.));
#63540=CARTESIAN_POINT('Origin',(20.5,0.,0.));
#63541=CARTESIAN_POINT('',(19.5,-9.,-1.10218211923262E-15));
#63542=CARTESIAN_POINT('Origin',(18.,18.5,0.));
#63543=CARTESIAN_POINT('',(18.,10.8187337521542,-14.3542676580869));
#63544=CARTESIAN_POINT('',(18.,11.4987322084552,-15.034266114388));
#63545=CARTESIAN_POINT('',(18.,9.32726009489054,-12.8627940008233));
#63546=CARTESIAN_POINT('',(18.,10.8518846384445,-14.9828768864291));
#63547=CARTESIAN_POINT('Origin',(18.,11.145178817862,-15.3878195049812));
#63548=CARTESIAN_POINT('',(18.,-10.8518846384445,-14.9828768864291));
#63549=CARTESIAN_POINT('Origin',(18.,0.,0.));
#63550=CARTESIAN_POINT('',(18.,-11.4987322084552,-15.034266114388));
#63551=CARTESIAN_POINT('Origin',(18.,-11.145178817862,-15.3878195049812));
#63552=CARTESIAN_POINT('',(18.,-10.8187337521542,-14.3542676580869));
#63553=CARTESIAN_POINT('',(18.,-0.501524163602491,-4.0370580695352));
#63554=CARTESIAN_POINT('',(18.,-14.3542676580869,-10.8187337521542));
#63555=CARTESIAN_POINT('',(18.,-7.07761722863737,-18.0953841816037));
#63556=CARTESIAN_POINT('',(18.,-15.034266114388,-11.4987322084552));
#63557=CARTESIAN_POINT('',(18.,-3.61279400082328,-0.0772600948905389));
#63558=CARTESIAN_POINT('',(18.,-14.9828768864291,-10.8518846384445));
#63559=CARTESIAN_POINT('Origin',(18.,-15.3878195049812,-11.145178817862));
#63560=CARTESIAN_POINT('',(18.,-18.5,-2.2655965784226E-15));
#63561=CARTESIAN_POINT('Origin',(18.,0.,0.));
#63562=CARTESIAN_POINT('',(18.,-14.9828768864291,10.8518846384445));
#63563=CARTESIAN_POINT('Origin',(18.,0.,0.));
#63564=CARTESIAN_POINT('',(18.,-15.034266114388,11.4987322084552));
#63565=CARTESIAN_POINT('Origin',(18.,-15.3878195049812,11.145178817862));
#63566=CARTESIAN_POINT('',(18.,-14.3542676580869,10.8187337521542));
#63567=CARTESIAN_POINT('',(18.,-4.03705806953519,0.501524163602477));
#63568=CARTESIAN_POINT('',(18.,-10.8187337521542,14.3542676580869));
#63569=CARTESIAN_POINT('',(18.,-8.84538418160373,16.3276172286374));
#63570=CARTESIAN_POINT('',(18.,-11.4987322084552,15.034266114388));
#63571=CARTESIAN_POINT('',(18.,-0.07726009489054,3.61279400082328));
#63572=CARTESIAN_POINT('',(18.,-10.8518846384445,14.9828768864291));
#63573=CARTESIAN_POINT('Origin',(18.,-11.145178817862,15.3878195049812));
#63574=CARTESIAN_POINT('',(18.,10.8518846384445,14.9828768864291));
#63575=CARTESIAN_POINT('Origin',(18.,0.,0.));
#63576=CARTESIAN_POINT('',(18.,11.4987322084552,15.034266114388));
#63577=CARTESIAN_POINT('Origin',(18.,11.145178817862,15.3878195049812));
#63578=CARTESIAN_POINT('',(18.,10.8187337521542,14.3542676580869));
#63579=CARTESIAN_POINT('',(18.,9.75152416360247,13.2870580695352));
#63580=CARTESIAN_POINT('',(18.,14.3542676580869,10.8187337521542));
#63581=CARTESIAN_POINT('',(18.,16.3276172286374,8.84538418160373));
#63582=CARTESIAN_POINT('',(18.,15.034266114388,11.4987322084552));
#63583=CARTESIAN_POINT('',(18.,12.8627940008233,9.32726009489054));
#63584=CARTESIAN_POINT('',(18.,14.9828768864291,10.8518846384445));
#63585=CARTESIAN_POINT('Origin',(18.,15.3878195049812,11.145178817862));
#63586=CARTESIAN_POINT('',(18.,14.9828768864291,-10.8518846384445));
#63587=CARTESIAN_POINT('Origin',(18.,0.,0.));
#63588=CARTESIAN_POINT('',(18.,15.034266114388,-11.4987322084552));
#63589=CARTESIAN_POINT('Origin',(18.,15.3878195049812,-11.145178817862));
#63590=CARTESIAN_POINT('',(18.,14.3542676580869,-10.8187337521542));
#63591=CARTESIAN_POINT('',(18.,13.2870580695352,-9.75152416360247));
#63592=CARTESIAN_POINT('',(18.,18.0953841816037,-7.07761722863736));
#63593=CARTESIAN_POINT('Origin',(20.5,0.,0.));
#63594=CARTESIAN_POINT('',(21.,-1.16341445918999E-15,9.5));
#63595=CARTESIAN_POINT('Origin',(20.5,-1.16341445918999E-15,9.5));
#63596=CARTESIAN_POINT('Origin',(21.,0.,0.));
#63597=CARTESIAN_POINT('Origin',(21.,9.,0.));
#63598=CARTESIAN_POINT('',(21.,14.3542676580869,-10.8187337521542));
#63599=CARTESIAN_POINT('',(21.,14.7292483497821,-11.1937144438494));
#63600=CARTESIAN_POINT('',(21.,10.9120580695352,-7.37652416360247));
#63601=CARTESIAN_POINT('',(21.,14.7292483497821,11.1937144438494));
#63602=CARTESIAN_POINT('Origin',(21.,0.,0.));
#63603=CARTESIAN_POINT('',(21.,14.3542676580869,10.8187337521542));
#63604=CARTESIAN_POINT('',(21.,10.4877940008233,6.95226009489054));
#63605=CARTESIAN_POINT('',(21.,10.8187337521542,14.3542676580869));
#63606=CARTESIAN_POINT('',(21.,13.9526172286374,11.2203841816037));
#63607=CARTESIAN_POINT('',(21.,11.1937144438494,14.7292483497821));
#63608=CARTESIAN_POINT('',(21.,7.37652416360247,10.9120580695352));
#63609=CARTESIAN_POINT('',(21.,-11.1937144438494,14.7292483497821));
#63610=CARTESIAN_POINT('Origin',(21.,0.,0.));
#63611=CARTESIAN_POINT('',(21.,-10.8187337521542,14.3542676580869));
#63612=CARTESIAN_POINT('',(21.,-2.45226009489054,5.98779400082328));
#63613=CARTESIAN_POINT('',(21.,-14.3542676580869,10.8187337521542));
#63614=CARTESIAN_POINT('',(21.,-11.2203841816037,13.9526172286374));
#63615=CARTESIAN_POINT('',(21.,-14.7292483497821,11.1937144438494));
#63616=CARTESIAN_POINT('',(21.,-6.41205806953519,2.87652416360248));
#63617=CARTESIAN_POINT('',(21.,-14.9828768864291,-10.8518846384445));
#63618=CARTESIAN_POINT('Origin',(21.,0.,0.));
#63619=CARTESIAN_POINT('',(21.,-15.034266114388,-11.4987322084552));
#63620=CARTESIAN_POINT('Origin',(21.,-15.3878195049812,-11.145178817862));
#63621=CARTESIAN_POINT('',(21.,-14.3542676580869,-10.8187337521542));
#63622=CARTESIAN_POINT('',(21.,-5.98779400082328,-2.45226009489054));
#63623=CARTESIAN_POINT('',(21.,-10.8187337521542,-14.3542676580869));
#63624=CARTESIAN_POINT('',(21.,-9.45261722863737,-15.7203841816037));
#63625=CARTESIAN_POINT('',(21.,-11.4987322084552,-15.034266114388));
#63626=CARTESIAN_POINT('',(21.,-2.87652416360248,-6.4120580695352));
#63627=CARTESIAN_POINT('',(21.,-10.8518846384445,-14.9828768864291));
#63628=CARTESIAN_POINT('Origin',(21.,-11.145178817862,-15.3878195049812));
#63629=CARTESIAN_POINT('',(21.,11.1937144438493,-14.7292483497821));
#63630=CARTESIAN_POINT('Origin',(21.,0.,0.));
#63631=CARTESIAN_POINT('',(21.,10.8187337521542,-14.3542676580869));
#63632=CARTESIAN_POINT('',(21.,6.95226009489054,-10.4877940008233));
#63633=CARTESIAN_POINT('',(21.,15.7203841816037,-9.45261722863736));
#63634=CARTESIAN_POINT('Origin',(18.5,18.0953841816037,-7.07761722863736));
#63635=CARTESIAN_POINT('',(18.5,14.7078210486802,-11.1722871427475));
#63636=CARTESIAN_POINT('Origin',(18.5,14.3542676580869,-10.8187337521542));
#63637=CARTESIAN_POINT('',(18.5,11.1722871427474,-14.7078210486802));
#63638=CARTESIAN_POINT('',(18.5,18.448937572197,-7.43117061923064));
#63639=CARTESIAN_POINT('Origin',(18.5,10.8187337521542,-14.3542676580869));
#63640=CARTESIAN_POINT('Origin',(8.,14.7078210486802,-11.1722871427475));
#63641=CARTESIAN_POINT('',(20.5,14.7078210486802,-11.1722871427475));
#63642=CARTESIAN_POINT('',(8.,14.7078210486802,-11.1722871427475));
#63643=CARTESIAN_POINT('',(20.5,11.1722871427474,-14.7078210486802));
#63644=CARTESIAN_POINT('',(20.5,16.073937572197,-9.80617061923064));
#63645=CARTESIAN_POINT('',(8.,11.1722871427474,-14.7078210486802));
#63646=CARTESIAN_POINT('Origin',(20.5,15.7203841816037,-9.45261722863736));
#63647=CARTESIAN_POINT('Origin',(20.5,10.8187337521542,-14.3542676580869));
#63648=CARTESIAN_POINT('Origin',(20.5,14.3542676580869,-10.8187337521542));
#63649=CARTESIAN_POINT('Origin',(18.5,16.3276172286374,8.84538418160373));
#63650=CARTESIAN_POINT('',(18.5,11.1722871427475,14.7078210486802));
#63651=CARTESIAN_POINT('Origin',(18.5,10.8187337521542,14.3542676580869));
#63652=CARTESIAN_POINT('',(18.5,14.7078210486802,11.1722871427475));
#63653=CARTESIAN_POINT('',(18.5,16.6811706192306,9.19893757219701));
#63654=CARTESIAN_POINT('Origin',(18.5,14.3542676580869,10.8187337521542));
#63655=CARTESIAN_POINT('Origin',(8.,11.1722871427475,14.7078210486802));
#63656=CARTESIAN_POINT('',(20.5,11.1722871427475,14.7078210486802));
#63657=CARTESIAN_POINT('',(8.,11.1722871427475,14.7078210486802));
#63658=CARTESIAN_POINT('',(20.5,14.7078210486802,11.1722871427475));
#63659=CARTESIAN_POINT('',(20.5,14.3061706192306,11.573937572197));
#63660=CARTESIAN_POINT('',(8.,14.7078210486802,11.1722871427475));
#63661=CARTESIAN_POINT('Origin',(20.5,13.9526172286374,11.2203841816037));
#63662=CARTESIAN_POINT('Origin',(20.5,14.3542676580869,10.8187337521542));
#63663=CARTESIAN_POINT('Origin',(20.5,10.8187337521542,14.3542676580869));
#63664=CARTESIAN_POINT('Origin',(18.5,-8.84538418160373,16.3276172286374));
#63665=CARTESIAN_POINT('',(18.5,-14.7078210486802,11.1722871427475));
#63666=CARTESIAN_POINT('Origin',(18.5,-14.3542676580869,10.8187337521542));
#63667=CARTESIAN_POINT('',(18.5,-11.1722871427475,14.7078210486802));
#63668=CARTESIAN_POINT('',(18.5,-9.198937572197,16.6811706192306));
#63669=CARTESIAN_POINT('Origin',(18.5,-10.8187337521542,14.3542676580869));
#63670=CARTESIAN_POINT('Origin',(8.,-14.7078210486802,11.1722871427475));
#63671=CARTESIAN_POINT('',(20.5,-14.7078210486802,11.1722871427475));
#63672=CARTESIAN_POINT('',(8.,-14.7078210486802,11.1722871427475));
#63673=CARTESIAN_POINT('',(20.5,-11.1722871427475,14.7078210486802));
#63674=CARTESIAN_POINT('',(20.5,-11.573937572197,14.3061706192306));
#63675=CARTESIAN_POINT('',(8.,-11.1722871427475,14.7078210486802));
#63676=CARTESIAN_POINT('Origin',(20.5,-11.2203841816037,13.9526172286374));
#63677=CARTESIAN_POINT('Origin',(20.5,-10.8187337521542,14.3542676580869));
#63678=CARTESIAN_POINT('Origin',(20.5,-14.3542676580869,10.8187337521542));
#63679=CARTESIAN_POINT('Origin',(-6.,0.,0.));
#63680=CARTESIAN_POINT('',(-6.5,-19.8947609985231,4.00000000022632));
#63681=CARTESIAN_POINT('',(-6.35355339174144,-20.2413779209503,4.0696900904913));
#63682=CARTESIAN_POINT('Origin',(-6.,-19.8947609985231,4.00000000022632));
#63683=CARTESIAN_POINT('',(-6.35355339174133,-4.06969009049129,20.2413779209503));
#63684=CARTESIAN_POINT('Origin',(-6.35355339059327,0.,0.));
#63685=CARTESIAN_POINT('',(-6.5,-4.,19.8947609985686));
#63686=CARTESIAN_POINT('Origin',(-6.,-4.0000000002263,19.8947609985231));
#63687=CARTESIAN_POINT('Origin',(-6.5,0.,0.));
#63688=CARTESIAN_POINT('Origin',(-6.,-4.,19.8947609985686));
#63689=CARTESIAN_POINT('',(-5.99999999557354,-3.5,19.8947610075986));
#63690=CARTESIAN_POINT('Origin',(-6.,-4.,19.8947609985686));
#63691=CARTESIAN_POINT('Origin',(-6.,-4.,19.8947609985686));
#63692=CARTESIAN_POINT('Origin',(-6.,1.25,4.));
#63693=CARTESIAN_POINT('',(-5.99999999549636,-19.8947610077561,3.5));
#63694=CARTESIAN_POINT('Origin',(-6.,-19.8947610077561,4.));
#63695=CARTESIAN_POINT('',(-6.5,-18.5741756210067,4.));
#63696=CARTESIAN_POINT('',(-6.5,1.25,4.));
#63697=CARTESIAN_POINT('',(-6.,-18.5741756210067,3.5));
#63698=CARTESIAN_POINT('Origin',(-6.,-18.5741756210067,4.));
#63699=CARTESIAN_POINT('',(-6.,1.25,3.5));
#63700=CARTESIAN_POINT('Origin',(-6.,-18.5741756210067,4.00000000000001));
#63701=CARTESIAN_POINT('',(-6.,-18.0853815257171,3.89473684210527));
#63702=CARTESIAN_POINT('Origin',(-6.,-18.5741756210067,4.00000000000001));
#63703=CARTESIAN_POINT('Origin',(-6.,-18.5741756210067,4.));
#63704=CARTESIAN_POINT('Origin',(-6.00000000002274,-19.8947609985454,4.));
#63705=CARTESIAN_POINT('Origin',(-6.00000000002274,-19.8947609985454,4.));
#63706=CARTESIAN_POINT('Origin',(-6.,-4.,10.75));
#63707=CARTESIAN_POINT('',(-6.,-3.5,18.5741756210067));
#63708=CARTESIAN_POINT('',(-6.,-3.5,10.75));
#63709=CARTESIAN_POINT('',(-6.5,-4.,18.5741756210067));
#63710=CARTESIAN_POINT('Origin',(-6.,-4.,18.5741756210067));
#63711=CARTESIAN_POINT('',(-6.5,-4.,10.75));
#63712=CARTESIAN_POINT('Ctrl Pts',(-6.3535533914602,-4.06969009037718,20.2413779206745));
#63713=CARTESIAN_POINT('Ctrl Pts',(-6.28452498011738,-4.0694530322025,20.3118353849912));
#63714=CARTESIAN_POINT('Ctrl Pts',(-6.21548931122258,-4.06921836800461,
20.3822849965481));
#63715=CARTESIAN_POINT('Ctrl Pts',(-6.14644660940672,-4.06898602743283,
20.4527269996664));
#63716=CARTESIAN_POINT('Ctrl Pts',(-6.36166082255246,-3.98902655650089,
20.2493262896997));
#63717=CARTESIAN_POINT('Ctrl Pts',(-6.29260192814692,-3.98880661885721,
20.3197549728352));
#63718=CARTESIAN_POINT('Ctrl Pts',(-6.22353638113495,-3.98858899315046,
20.3901763349667));
#63719=CARTESIAN_POINT('Ctrl Pts',(-6.15446386581863,-3.98837349192522,
20.4605901563));
#63720=CARTESIAN_POINT('Ctrl Pts',(-6.34907271559258,-3.82240661064016,
20.2369851525001));
#63721=CARTESIAN_POINT('Ctrl Pts',(-6.2799695713994,-3.82224326499387,20.3073687547676));
#63722=CARTESIAN_POINT('Ctrl Pts',(-6.21086028406924,-3.82208099151617,
20.3777455503893));
#63723=CARTESIAN_POINT('Ctrl Pts',(-6.14174450682076,-3.82192100742865,
20.4481152762486));
#63724=CARTESIAN_POINT('Ctrl Pts',(-6.23193279948825,-3.5782931243035,20.1221434387457));
#63725=CARTESIAN_POINT('Ctrl Pts',(-6.16282464783201,-3.57824724809786,
20.1925063334978));
#63726=CARTESIAN_POINT('Ctrl Pts',(-6.09371017517293,-3.57820215914787,
20.2628625082749));
#63727=CARTESIAN_POINT('Ctrl Pts',(-6.02458951791509,-3.57815724852431,
20.3332121247398));
#63728=CARTESIAN_POINT('Ctrl Pts',(-6.08725162138116,-3.5,19.9803008030806));
#63729=CARTESIAN_POINT('Ctrl Pts',(-6.01819267795923,-3.50000086638446,
20.0506924552528));
#63730=CARTESIAN_POINT('Ctrl Pts',(-5.94912751000377,-3.49999915309731,
20.1210777460986));
#63731=CARTESIAN_POINT('Ctrl Pts',(-5.88005496058486,-3.5,20.1914556678078));
#63732=CARTESIAN_POINT('Ctrl Pts',(-6.00000000086693,-3.5,19.8947609976843));
#63733=CARTESIAN_POINT('Ctrl Pts',(-5.9309715895241,-3.5,19.9651707995687));
#63734=CARTESIAN_POINT('Ctrl Pts',(-5.8619359206293,-3.5,20.0355734829672));
#63735=CARTESIAN_POINT('Ctrl Pts',(-5.79289321881344,-3.5,20.1059692628831));
#63736=CARTESIAN_POINT('',(-6.14644660940672,-4.06898602743283,20.4527269996663));
#63737=CARTESIAN_POINT('Ctrl Pts',(-6.3535533914602,-4.06969009037718,20.2413779206745));
#63738=CARTESIAN_POINT('Ctrl Pts',(-6.28452498011738,-4.0694530322025,20.3118353849912));
#63739=CARTESIAN_POINT('Ctrl Pts',(-6.21548931122258,-4.06921836800461,
20.3822849965481));
#63740=CARTESIAN_POINT('Ctrl Pts',(-6.14644660940672,-4.06898602743283,
20.4527269996664));
#63741=CARTESIAN_POINT('',(-5.79289321881344,-3.5,20.1059692628831));
#63742=CARTESIAN_POINT('Origin',(-5.79289321881344,-4.,20.1059692628831));
#63743=CARTESIAN_POINT('Ctrl Pts',(-5.79289321881344,-3.5,20.1059692628831));
#63744=CARTESIAN_POINT('Ctrl Pts',(-5.86193591811196,-3.5,20.0355734855339));
#63745=CARTESIAN_POINT('Ctrl Pts',(-5.93097158448994,-3.5,19.9651708047025));
#63746=CARTESIAN_POINT('Ctrl Pts',(-5.99999999331647,-3.5,19.8947610053858));
#63747=CARTESIAN_POINT('Origin',(-6.25,0.,0.));
#63748=CARTESIAN_POINT('',(-6.14644660940672,-20.4527269996663,4.06898602743284));
#63749=CARTESIAN_POINT('Ctrl Pts',(-6.14644660940672,-20.4527269996663,
4.06898602743284));
#63750=CARTESIAN_POINT('Ctrl Pts',(-6.21548931371643,-20.3822849940037,
4.06921836801301));
#63751=CARTESIAN_POINT('Ctrl Pts',(-6.28452498219244,-20.3118353828732,
4.06945303220963));
#63752=CARTESIAN_POINT('Ctrl Pts',(-6.35355339146028,-20.2413779206745,
4.06969009037718));
#63753=CARTESIAN_POINT('Origin',(-6.14644660940672,-1.11022302462516E-15,
-1.11022302462516E-15));
#63754=CARTESIAN_POINT('Ctrl Pts',(-6.000000000867,-19.8947609976842,3.5));
#63755=CARTESIAN_POINT('Ctrl Pts',(-5.93097159159917,-19.9651707974521,
3.5));
#63756=CARTESIAN_POINT('Ctrl Pts',(-5.86193592312316,-20.0355734804245,
3.5));
#63757=CARTESIAN_POINT('Ctrl Pts',(-5.79289321881345,-20.1059692628831,
3.5));
#63758=CARTESIAN_POINT('Ctrl Pts',(-6.05816774787649,-19.9517875346151,
3.5));
#63759=CARTESIAN_POINT('Ctrl Pts',(-5.98911910175446,-20.0221853405778,
3.50000009695088));
#63760=CARTESIAN_POINT('Ctrl Pts',(-5.92006353441284,-20.0925762189771,
3.49999990514108));
#63761=CARTESIAN_POINT('Ctrl Pts',(-5.85100104666106,-20.1629601994995,
3.5));
#63762=CARTESIAN_POINT('Ctrl Pts',(-6.17423130885212,-20.0655740105676,
3.54067994796965));
#63763=CARTESIAN_POINT('Ctrl Pts',(-6.10514245467535,-20.1359480599334,
3.5406567970824));
#63764=CARTESIAN_POINT('Ctrl Pts',(-6.03604760619308,-20.2063157855124,
3.5406339242176));
#63765=CARTESIAN_POINT('Ctrl Pts',(-5.96694581109642,-20.2766763882766,
3.5406112586698));
#63766=CARTESIAN_POINT('Ctrl Pts',(-6.33051862773969,-20.2187950827352,
3.73714712174979));
#63767=CARTESIAN_POINT('Ctrl Pts',(-6.26140157368465,-20.2891625274127,
3.73702083787885));
#63768=CARTESIAN_POINT('Ctrl Pts',(-6.19227807841401,-20.359522954417,3.73689570997189));
#63769=CARTESIAN_POINT('Ctrl Pts',(-6.12314870346812,-20.4298769030473,
3.73677204602557));
#63770=CARTESIAN_POINT('Ctrl Pts',(-6.36571453809866,-20.2533004742123,
3.94869478956275));
#63771=CARTESIAN_POINT('Ctrl Pts',(-6.29663981942388,-20.3237142523843,
3.94848324312937));
#63772=CARTESIAN_POINT('Ctrl Pts',(-6.22756048974816,-20.394122502803,3.94827446993852));
#63773=CARTESIAN_POINT('Ctrl Pts',(-6.1584724940246,-20.4645217346169,3.94806722417142));
#63774=CARTESIAN_POINT('Ctrl Pts',(-6.35355339146028,-20.2413779206745,
4.06969009037718));
#63775=CARTESIAN_POINT('Ctrl Pts',(-6.28452498219244,-20.3118353828732,
4.06945303220963));
#63776=CARTESIAN_POINT('Ctrl Pts',(-6.21548931371643,-20.3822849940037,
4.06921836801301));
#63777=CARTESIAN_POINT('Ctrl Pts',(-6.14644660940672,-20.4527269996663,
4.06898602743284));
#63778=CARTESIAN_POINT('',(-5.79289321881345,-20.1059692628831,3.5));
#63779=CARTESIAN_POINT('Ctrl Pts',(-5.99999999319992,-19.8947610055047,
3.5));
#63780=CARTESIAN_POINT('Ctrl Pts',(-5.93097158648724,-19.9651708026652,
3.5));
#63781=CARTESIAN_POINT('Ctrl Pts',(-5.86193592056693,-20.0355734830308,
3.5));
#63782=CARTESIAN_POINT('Ctrl Pts',(-5.79289321881345,-20.1059692628831,
3.5));
#63783=CARTESIAN_POINT('Origin',(-5.79289321881345,-20.1059692628831,4.));
#63784=CARTESIAN_POINT('Origin',(-6.5,-18.,3.5));
#63785=CARTESIAN_POINT('',(-2.49011275698595,-18.5741756210067,3.5));
#63786=CARTESIAN_POINT('',(5.75,-18.5741756210067,3.5));
#63787=CARTESIAN_POINT('',(-2.5,-18.6748493969831,3.5));
#63788=CARTESIAN_POINT('Ctrl Pts',(-2.5,-18.6748493969831,3.5));
#63789=CARTESIAN_POINT('Ctrl Pts',(-2.5,-18.643018830074,3.5));
#63790=CARTESIAN_POINT('Ctrl Pts',(-2.49686768006346,-18.608225302467,3.5));
#63791=CARTESIAN_POINT('Ctrl Pts',(-2.49011275698578,-18.5741756210058,
3.5));
#63792=CARTESIAN_POINT('',(-2.5,-20.1059692628831,3.5));
#63793=CARTESIAN_POINT('',(-2.5,-18.,3.5));
#63794=CARTESIAN_POINT('',(11.6,-20.1059692628831,3.5));
#63795=CARTESIAN_POINT('Origin',(11.6,-20.1059692628831,4.));
#63796=CARTESIAN_POINT('',(-2.,-20.5963587570998,4.09756097560976));
#63797=CARTESIAN_POINT('',(-2.5,-20.1975426238546,3.50845720475184));
#63798=CARTESIAN_POINT('Ctrl Pts',(-2.,-20.5963587570998,4.09756097560976));
#63799=CARTESIAN_POINT('Ctrl Pts',(-2.0007819915549,-20.5965131903849,4.09678471788856));
#63800=CARTESIAN_POINT('Ctrl Pts',(-2.00156398410941,-20.5966657807117,
4.09600809248874));
#63801=CARTESIAN_POINT('Ctrl Pts',(-2.05717822849771,-20.6073867069003,
4.04074949570648));
#63802=CARTESIAN_POINT('Ctrl Pts',(-2.11233881531681,-20.6089573942057,
3.98414057845334));
#63803=CARTESIAN_POINT('Ctrl Pts',(-2.21839474851504,-20.5925290379239,
3.87165457010946));
#63804=CARTESIAN_POINT('Ctrl Pts',(-2.2700758750267,-20.5745079871765,3.81496483783112));
#63805=CARTESIAN_POINT('Ctrl Pts',(-2.3578137004182,-20.5197688252063,3.71434799515287));
#63806=CARTESIAN_POINT('Ctrl Pts',(-2.39549276964077,-20.4855489795038,
3.66919971187174));
#63807=CARTESIAN_POINT('Ctrl Pts',(-2.45004388530638,-20.4077033015026,
3.59868523815613));
#63808=CARTESIAN_POINT('Ctrl Pts',(-2.46954638452372,-20.3681432457135,
3.57134136668746));
#63809=CARTESIAN_POINT('Ctrl Pts',(-2.49393578234053,-20.2839850074225,
3.53073227474396));
#63810=CARTESIAN_POINT('Ctrl Pts',(-2.49999999999998,-20.2417646390697,
3.51669567066231));
#63811=CARTESIAN_POINT('Ctrl Pts',(-2.5,-20.1975426238548,3.50845720475187));
#63812=CARTESIAN_POINT('',(-5.79289321881345,-20.5963587570998,4.09756097560976));
#63813=CARTESIAN_POINT('',(11.6,-20.5963587570998,4.09756097560976));
#63814=CARTESIAN_POINT('Origin',(-5.79289321881345,-20.1059692628831,4.));
#63815=CARTESIAN_POINT('Origin',(-2.5,-20.1059692628831,4.));
#63816=CARTESIAN_POINT('Origin',(-5.79289321881345,-20.1059692628831,4.));
#63817=CARTESIAN_POINT('Origin',(-5.79289321881345,-20.1059692628831,4.));
#63818=CARTESIAN_POINT('Origin',(-6.5,20.5,0.));
#63819=CARTESIAN_POINT('Origin',(-6.5,0.,0.));
#63820=CARTESIAN_POINT('Origin',(-5.79289321881345,0.,0.));
#63821=CARTESIAN_POINT('',(-5.79289321881344,-4.09756097560975,20.5963587570998));
#63822=CARTESIAN_POINT('Origin',(-5.79289321881345,0.,0.));
#63823=CARTESIAN_POINT('Origin',(-5.79289321881344,-4.,20.1059692628831));
#63824=CARTESIAN_POINT('Origin',(11.6,0.,0.));
#63825=CARTESIAN_POINT('',(28.9928932188134,-21.,-2.57175827820944E-15));
#63826=CARTESIAN_POINT('',(28.9928932188134,-2.57175827820944E-15,21.));
#63827=CARTESIAN_POINT('Origin',(28.9928932188134,0.,0.));
#63828=CARTESIAN_POINT('',(-2.,-21.,-2.57175827820944E-15));
#63829=CARTESIAN_POINT('',(11.6,-21.,-2.57175827820944E-15));
#63830=CARTESIAN_POINT('',(-2.,-20.5963587570998,-4.09756097560975));
#63831=CARTESIAN_POINT('Origin',(-2.,0.,0.));
#63832=CARTESIAN_POINT('',(-6.,-20.5963587570998,-4.09756097560975));
#63833=CARTESIAN_POINT('',(11.6,-20.5963587570998,-4.09756097560975));
#63834=CARTESIAN_POINT('',(-6.,-4.09756097560976,-20.5963587570998));
#63835=CARTESIAN_POINT('Origin',(-6.,0.,0.));
#63836=CARTESIAN_POINT('',(-2.,-4.09756097560976,-20.5963587570998));
#63837=CARTESIAN_POINT('',(11.6,-4.09756097560976,-20.5963587570998));
#63838=CARTESIAN_POINT('',(-2.,4.09756097560975,-20.5963587570998));
#63839=CARTESIAN_POINT('Origin',(-2.,0.,0.));
#63840=CARTESIAN_POINT('',(-5.79289321881345,4.09756097560975,-20.5963587570998));
#63841=CARTESIAN_POINT('',(11.6,4.09756097560975,-20.5963587570998));
#63842=CARTESIAN_POINT('',(-5.79289321881345,20.5963587570998,-4.09756097560975));
#63843=CARTESIAN_POINT('Origin',(-5.79289321881345,0.,0.));
#63844=CARTESIAN_POINT('',(-2.,20.5963587570998,-4.09756097560975));
#63845=CARTESIAN_POINT('',(11.6,20.5963587570998,-4.09756097560975));
#63846=CARTESIAN_POINT('',(-2.,20.5963587570998,4.09756097560975));
#63847=CARTESIAN_POINT('Origin',(-2.,0.,0.));
#63848=CARTESIAN_POINT('',(-5.79289321881345,20.5963587570998,4.09756097560976));
#63849=CARTESIAN_POINT('',(11.6,20.5963587570998,4.09756097560975));
#63850=CARTESIAN_POINT('',(-5.79289321881345,4.09756097560976,20.5963587570998));
#63851=CARTESIAN_POINT('Origin',(-5.79289321881345,0.,0.));
#63852=CARTESIAN_POINT('',(-2.,4.09756097560976,20.5963587570998));
#63853=CARTESIAN_POINT('',(11.6,4.09756097560976,20.5963587570998));
#63854=CARTESIAN_POINT('',(-2.,-4.09756097560976,20.5963587570998));
#63855=CARTESIAN_POINT('Origin',(-2.,0.,0.));
#63856=CARTESIAN_POINT('',(11.6,-4.09756097560975,20.5963587570998));
#63857=CARTESIAN_POINT('Origin',(-2.,0.,0.));
#63858=CARTESIAN_POINT('Origin',(28.9928932188134,0.,0.));
#63859=CARTESIAN_POINT('Origin',(11.6,20.1059692628831,4.));
#63860=CARTESIAN_POINT('',(-2.5,20.1975426238546,3.50845720475184));
#63861=CARTESIAN_POINT('',(-2.5,20.1059692628831,3.5));
#63862=CARTESIAN_POINT('Origin',(-2.5,20.1059692628831,4.));
#63863=CARTESIAN_POINT('',(-5.79289321881345,20.1059692628831,3.5));
#63864=CARTESIAN_POINT('',(11.6,20.1059692628831,3.5));
#63865=CARTESIAN_POINT('Origin',(-5.79289321881345,20.1059692628831,4.));
#63866=CARTESIAN_POINT('Ctrl Pts',(-2.5,20.1975426238546,3.50845720475184));
#63867=CARTESIAN_POINT('Ctrl Pts',(-2.5,20.2417646390367,3.51669567065614));
#63868=CARTESIAN_POINT('Ctrl Pts',(-2.49393578234954,20.2839850073609,3.5307322747233));
#63869=CARTESIAN_POINT('Ctrl Pts',(-2.46954638455826,20.3681432456292,3.5713413666364));
#63870=CARTESIAN_POINT('Ctrl Pts',(-2.45004388535121,20.4077033014208,3.59868523809492));
#63871=CARTESIAN_POINT('Ctrl Pts',(-2.39549276970982,20.4855489794284,3.66919971178668));
#63872=CARTESIAN_POINT('Ctrl Pts',(-2.35781370050222,20.5197688251367,3.71434799505337));
#63873=CARTESIAN_POINT('Ctrl Pts',(-2.27007587511498,20.5745079871413,3.81496483773348));
#63874=CARTESIAN_POINT('Ctrl Pts',(-2.21839474858771,20.5925290379056,3.87165457003106));
#63875=CARTESIAN_POINT('Ctrl Pts',(-2.11233881535515,20.6089573942069,3.98414057841399));
#63876=CARTESIAN_POINT('Ctrl Pts',(-2.05717822853915,20.6073867068998,4.04074949570797));
#63877=CARTESIAN_POINT('Ctrl Pts',(-2.00156398410875,20.5966657807121,4.09600809248684));
#63878=CARTESIAN_POINT('Ctrl Pts',(-2.00078199155489,20.5965131903849,4.09678471788857));
#63879=CARTESIAN_POINT('Ctrl Pts',(-2.,20.5963587570998,4.09756097560976));
#63880=CARTESIAN_POINT('Origin',(-5.79289321881345,20.1059692628831,4.));
#63881=CARTESIAN_POINT('',(-6.14644660940673,20.4527269996663,4.06898602743283));
#63882=CARTESIAN_POINT('Origin',(-5.79289321881345,20.1059692628831,4.));
#63883=CARTESIAN_POINT('Origin',(-5.79289321881345,20.1059692628831,4.));
#63884=CARTESIAN_POINT('Origin',(-6.,19.8947609985686,4.));
#63885=CARTESIAN_POINT('',(-6.35355339059328,20.2413779215594,4.0696900903742));
#63886=CARTESIAN_POINT('',(-6.,19.8947609985686,3.5));
#63887=CARTESIAN_POINT('Origin',(-6.,19.8947609985686,4.));
#63888=CARTESIAN_POINT('',(-6.5,19.8947609985686,4.));
#63889=CARTESIAN_POINT('Origin',(-6.,19.8947609985686,4.));
#63890=CARTESIAN_POINT('Origin',(-6.,19.8947609985686,4.));
#63891=CARTESIAN_POINT('Ctrl Pts',(-6.35355339059328,20.2413779215594,4.0696900903742));
#63892=CARTESIAN_POINT('Ctrl Pts',(-6.28452498165401,20.3118353834226,4.0694530322078));
#63893=CARTESIAN_POINT('Ctrl Pts',(-6.21548931347971,20.3822849942452,4.06921836801221));
#63894=CARTESIAN_POINT('Ctrl Pts',(-6.14644660940673,20.4527269996663,4.06898602743283));
#63895=CARTESIAN_POINT('Ctrl Pts',(-6.36166082168515,20.2493262905843,3.98902655649813));
#63896=CARTESIAN_POINT('Ctrl Pts',(-6.29260192968424,20.3197549712672,3.98880661886213));
#63897=CARTESIAN_POINT('Ctrl Pts',(-6.22353638339306,20.3901763326647,3.98858899315751));
#63898=CARTESIAN_POINT('Ctrl Pts',(-6.15446386581864,20.4605901563,3.98837349192522));
#63899=CARTESIAN_POINT('Ctrl Pts',(-6.34907271472472,20.2369851533841,3.8224066106381));
#63900=CARTESIAN_POINT('Ctrl Pts',(-6.27996957293771,20.3073687532007,3.82224326499752));
#63901=CARTESIAN_POINT('Ctrl Pts',(-6.21086028632876,20.3777455480888,3.82208099152141));
#63902=CARTESIAN_POINT('Ctrl Pts',(-6.14174450682077,20.4481152762486,3.82192100742866));
#63903=CARTESIAN_POINT('Ctrl Pts',(-6.23193279862033,20.1221434396294,3.57829312430292));
#63904=CARTESIAN_POINT('Ctrl Pts',(-6.16282464937043,20.1925063319313,3.57824724809889));
#63905=CARTESIAN_POINT('Ctrl Pts',(-6.09371017743262,20.2628625059751,3.57820215914935));
#63906=CARTESIAN_POINT('Ctrl Pts',(-6.02458951791509,20.3332121247397,3.57815724852431));
#63907=CARTESIAN_POINT('Ctrl Pts',(-6.08725162051385,19.9803008039646,3.5));
#63908=CARTESIAN_POINT('Ctrl Pts',(-6.01819267949655,20.0506924536857,3.50000086638443));
#63909=CARTESIAN_POINT('Ctrl Pts',(-5.94912751226188,20.1210777437978,3.49999915309729));
#63910=CARTESIAN_POINT('Ctrl Pts',(-5.88005496058487,20.1914556678078,3.5));
#63911=CARTESIAN_POINT('Ctrl Pts',(-6.,19.8947609985686,3.5));
#63912=CARTESIAN_POINT('Ctrl Pts',(-5.93097159106074,19.9651707980012,3.5));
#63913=CARTESIAN_POINT('Ctrl Pts',(-5.86193592288644,20.0355734806659,3.5));
#63914=CARTESIAN_POINT('Ctrl Pts',(-5.79289321881345,20.1059692628831,3.5));
#63915=CARTESIAN_POINT('Ctrl Pts',(-6.35355339059328,20.2413779215594,4.0696900903742));
#63916=CARTESIAN_POINT('Ctrl Pts',(-6.28452498165401,20.3118353834226,4.0694530322078));
#63917=CARTESIAN_POINT('Ctrl Pts',(-6.21548931347971,20.3822849942452,4.06921836801221));
#63918=CARTESIAN_POINT('Ctrl Pts',(-6.14644660940673,20.4527269996663,4.06898602743283));
#63919=CARTESIAN_POINT('Ctrl Pts',(-5.79289321881345,20.1059692628831,3.5));
#63920=CARTESIAN_POINT('Ctrl Pts',(-5.86193592288644,20.0355734806659,3.5));
#63921=CARTESIAN_POINT('Ctrl Pts',(-5.93097159106074,19.9651707980012,3.5));
#63922=CARTESIAN_POINT('Ctrl Pts',(-6.,19.8947609985686,3.5));
#63923=CARTESIAN_POINT('Origin',(-5.79289321881345,0.,0.));
#63924=CARTESIAN_POINT('',(-6.14644665398816,4.06898603193227,20.4527269760436));
#63925=CARTESIAN_POINT('Origin',(-6.14644660940673,1.11022302462516E-15,
0.));
#63926=CARTESIAN_POINT('Origin',(-5.79289321881345,4.,20.1059692628831));
#63927=CARTESIAN_POINT('Origin',(-6.25,0.,0.));
#63928=CARTESIAN_POINT('',(-6.35355339059327,4.0696900903742,20.2413779215594));
#63929=CARTESIAN_POINT('Origin',(-6.35355339059328,1.11022302462516E-15,
0.));
#63930=CARTESIAN_POINT('Ctrl Pts',(-6.14644664306266,4.06898602754609,20.4527269653283));
#63931=CARTESIAN_POINT('Ctrl Pts',(-6.21548933585545,4.06921836808827,20.3822849714111));
#63932=CARTESIAN_POINT('Ctrl Pts',(-6.28452499284272,4.06945303224623,20.3118353720023));
#63933=CARTESIAN_POINT('Ctrl Pts',(-6.35355339059327,4.0696900903742,20.2413779215594));
#63934=CARTESIAN_POINT('Origin',(-6.,0.,0.));
#63935=CARTESIAN_POINT('',(-6.5,4.,19.8947609985686));
#63936=CARTESIAN_POINT('Origin',(-6.5,0.,0.));
#63937=CARTESIAN_POINT('Origin',(-6.,4.,19.8947609985686));
#63938=CARTESIAN_POINT('Origin',(-2.,0.,0.));
#63939=CARTESIAN_POINT('',(-2.5,20.1975426238546,-3.50845720475184));
#63940=CARTESIAN_POINT('Ctrl Pts',(-2.5,20.1975426238546,-3.50845720475184));
#63941=CARTESIAN_POINT('Ctrl Pts',(-2.5,20.2435547744773,-3.51702916902183));
#63942=CARTESIAN_POINT('Ctrl Pts',(-2.49343634644932,20.2873343735479,-3.53186471227266));
#63943=CARTESIAN_POINT('Ctrl Pts',(-2.46720605754511,20.3741519147674,-3.57485564306978));
#63944=CARTESIAN_POINT('Ctrl Pts',(-2.44629528850599,20.414637889374,-3.60381971113445));
#63945=CARTESIAN_POINT('Ctrl Pts',(-2.38730845067544,20.4946845355157,-3.67931541228553));
#63946=CARTESIAN_POINT('Ctrl Pts',(-2.3460988108993,20.529374025357,-3.72819973354602));
#63947=CARTESIAN_POINT('Ctrl Pts',(-2.25735953173236,20.5791609950881,-3.82895180434606));
#63948=CARTESIAN_POINT('Ctrl Pts',(-2.20924193430928,20.5945414427225,-3.88147391652599));
#63949=CARTESIAN_POINT('Ctrl Pts',(-2.10884374679329,20.6088074165326,-3.98771778608995));
#63950=CARTESIAN_POINT('Ctrl Pts',(-2.05580187972944,20.6070466944948,-4.0421021986681));
#63951=CARTESIAN_POINT('Ctrl Pts',(-2.0020305645695,20.5967566605905,-4.09554468173573));
#63952=CARTESIAN_POINT('Ctrl Pts',(-2.00101528119124,20.5965592620908,-4.09655313881285));
#63953=CARTESIAN_POINT('Ctrl Pts',(-2.,20.5963587570998,-4.09756097560975));
#63954=CARTESIAN_POINT('Origin',(-2.5,0.,0.));
#63955=CARTESIAN_POINT('Origin',(-2.5,19.75,0.));
#63956=CARTESIAN_POINT('',(-2.5,20.1059692628831,-3.5));
#63957=CARTESIAN_POINT('Origin',(-2.5,20.1059692628831,-4.));
#63958=CARTESIAN_POINT('',(-2.5,18.6748493969831,-3.5));
#63959=CARTESIAN_POINT('',(-2.5,18.,-3.5));
#63960=CARTESIAN_POINT('',(-2.5,18.6748493969831,3.5));
#63961=CARTESIAN_POINT('Origin',(-2.5,0.,0.));
#63962=CARTESIAN_POINT('',(-2.5,21.5,3.5));
#63963=CARTESIAN_POINT('Origin',(-6.,3.99999999999999,-19.8947609985686));
#63964=CARTESIAN_POINT('',(-6.35355339059327,4.06969009037419,-20.2413779215594));
#63965=CARTESIAN_POINT('',(-6.,3.5,-19.8947609985686));
#63966=CARTESIAN_POINT('Origin',(-6.,3.99999999999999,-19.8947609985686));
#63967=CARTESIAN_POINT('',(-6.5,4.,-19.8947609985686));
#63968=CARTESIAN_POINT('Origin',(-6.,4.,-19.8947609985686));
#63969=CARTESIAN_POINT('Origin',(-6.,3.99999999999999,-19.8947609985686));
#63970=CARTESIAN_POINT('Origin',(-5.79289321881345,0.,0.));
#63971=CARTESIAN_POINT('',(-6.14644660940673,4.06898602743283,-20.4527269996663));
#63972=CARTESIAN_POINT('Origin',(-5.79289321881345,4.,-20.1059692628831));
#63973=CARTESIAN_POINT('',(-6.14644660940673,20.4527269996663,-4.06898602743283));
#63974=CARTESIAN_POINT('Origin',(-6.14644660940673,-1.11022302462516E-15,
-1.11022302462516E-15));
#63975=CARTESIAN_POINT('Origin',(-5.79289321881345,20.1059692628831,-4.));
#63976=CARTESIAN_POINT('Origin',(-5.79289321881345,4.,-20.1059692628831));
#63977=CARTESIAN_POINT('',(-5.79289321881345,3.5,-20.1059692628831));
#63978=CARTESIAN_POINT('Origin',(-5.79289321881345,4.,-20.1059692628831));
#63979=CARTESIAN_POINT('Origin',(-5.79289321881345,4.,-20.1059692628831));
#63980=CARTESIAN_POINT('Origin',(-5.79289321881345,20.1059692628831,-4.));
#63981=CARTESIAN_POINT('',(-5.79289321881345,20.1059692628831,-3.5));
#63982=CARTESIAN_POINT('Origin',(-5.79289321881345,20.1059692628831,-4.));
#63983=CARTESIAN_POINT('Origin',(-5.79289321881345,20.1059692628831,-4.));
#63984=CARTESIAN_POINT('Origin',(-6.,19.8947609985686,-4.));
#63985=CARTESIAN_POINT('',(-6.,19.8947609985686,-3.5));
#63986=CARTESIAN_POINT('',(-6.35355339059327,20.2413779215594,-4.0696900903742));
#63987=CARTESIAN_POINT('Origin',(-6.,19.8947609985686,-4.));
#63988=CARTESIAN_POINT('',(-6.5,19.8947609985686,-4.));
#63989=CARTESIAN_POINT('Origin',(-6.,19.8947609985686,-4.));
#63990=CARTESIAN_POINT('Origin',(-6.,19.8947609985686,-4.));
#63991=CARTESIAN_POINT('Ctrl Pts',(-6.14644660940673,20.4527269996663,-4.06898602743283));
#63992=CARTESIAN_POINT('Ctrl Pts',(-6.21548931338964,20.3822849943371,-4.06921836801191));
#63993=CARTESIAN_POINT('Ctrl Pts',(-6.28452498159193,20.311835383486,-4.06945303220759));
#63994=CARTESIAN_POINT('Ctrl Pts',(-6.35355339059328,20.2413779215594,-4.0696900903742));
#63995=CARTESIAN_POINT('Ctrl Pts',(-6.15446386581864,20.4605901563,-3.98837349192522));
#63996=CARTESIAN_POINT('Ctrl Pts',(-6.22353638330296,20.3901763327566,-3.98858899315722));
#63997=CARTESIAN_POINT('Ctrl Pts',(-6.29260192962212,20.3197549713306,-3.98880661886193));
#63998=CARTESIAN_POINT('Ctrl Pts',(-6.36166082168515,20.2493262905843,-3.98902655649813));
#63999=CARTESIAN_POINT('Ctrl Pts',(-6.14174450682077,20.4481152762486,-3.82192100742866));
#64000=CARTESIAN_POINT('Ctrl Pts',(-6.21086028623859,20.3777455481806,-3.8220809915212));
#64001=CARTESIAN_POINT('Ctrl Pts',(-6.27996957287556,20.307368753264,-3.82224326499737));
#64002=CARTESIAN_POINT('Ctrl Pts',(-6.34907271472472,20.2369851533841,-3.8224066106381));
#64003=CARTESIAN_POINT('Ctrl Pts',(-6.02458951791509,20.3332121247397,-3.57815724852431));
#64004=CARTESIAN_POINT('Ctrl Pts',(-6.09371017734244,20.2628625060668,-3.57820215914929));
#64005=CARTESIAN_POINT('Ctrl Pts',(-6.16282464930827,20.1925063319946,-3.57824724809885));
#64006=CARTESIAN_POINT('Ctrl Pts',(-6.23193279862033,20.1221434396294,-3.57829312430293));
#64007=CARTESIAN_POINT('Ctrl Pts',(-5.88005496058487,20.1914556678078,-3.5));
#64008=CARTESIAN_POINT('Ctrl Pts',(-5.94912751217177,20.1210777438896,-3.49999915309729));
#64009=CARTESIAN_POINT('Ctrl Pts',(-6.01819267943444,20.0506924537491,-3.50000086638443));
#64010=CARTESIAN_POINT('Ctrl Pts',(-6.08725162051385,19.9803008039646,-3.5));
#64011=CARTESIAN_POINT('Ctrl Pts',(-5.79289321881345,20.1059692628831,-3.5));
#64012=CARTESIAN_POINT('Ctrl Pts',(-5.86193592279637,20.0355734807577,-3.5));
#64013=CARTESIAN_POINT('Ctrl Pts',(-5.93097159099865,19.9651707980645,-3.5));
#64014=CARTESIAN_POINT('Ctrl Pts',(-6.,19.8947609985686,-3.5));
#64015=CARTESIAN_POINT('Ctrl Pts',(-6.,19.8947609985686,-3.5));
#64016=CARTESIAN_POINT('Ctrl Pts',(-5.93097159099865,19.9651707980645,-3.5));
#64017=CARTESIAN_POINT('Ctrl Pts',(-5.86193592279637,20.0355734807577,-3.5));
#64018=CARTESIAN_POINT('Ctrl Pts',(-5.79289321881345,20.1059692628831,-3.5));
#64019=CARTESIAN_POINT('Ctrl Pts',(-6.14644660940673,20.4527269996663,-4.06898602743283));
#64020=CARTESIAN_POINT('Ctrl Pts',(-6.21548931338964,20.3822849943371,-4.06921836801191));
#64021=CARTESIAN_POINT('Ctrl Pts',(-6.28452498159193,20.311835383486,-4.06945303220759));
#64022=CARTESIAN_POINT('Ctrl Pts',(-6.35355339059328,20.2413779215594,-4.0696900903742));
#64023=CARTESIAN_POINT('Ctrl Pts',(-6.35355339059328,4.0696900903742,-20.2413779215594));
#64024=CARTESIAN_POINT('Ctrl Pts',(-6.28452498163503,4.06945303220773,-20.311835383442));
#64025=CARTESIAN_POINT('Ctrl Pts',(-6.2154893134119,4.06921836801198,-20.3822849943144));
#64026=CARTESIAN_POINT('Ctrl Pts',(-6.14644660940672,4.06898602743283,-20.4527269996663));
#64027=CARTESIAN_POINT('Ctrl Pts',(-6.36166082168515,3.98902655649812,-20.2493262905843));
#64028=CARTESIAN_POINT('Ctrl Pts',(-6.29260192966524,3.98880661886206,-20.3197549712866));
#64029=CARTESIAN_POINT('Ctrl Pts',(-6.22353638332523,3.98858899315729,-20.3901763327339));
#64030=CARTESIAN_POINT('Ctrl Pts',(-6.15446386581864,3.98837349192522,-20.4605901563));
#64031=CARTESIAN_POINT('Ctrl Pts',(-6.34907271472472,3.8224066106381,-20.2369851533841));
#64032=CARTESIAN_POINT('Ctrl Pts',(-6.2799695729187,3.82224326499747,-20.30736875322));
#64033=CARTESIAN_POINT('Ctrl Pts',(-6.21086028626087,3.82208099152124,-20.3777455481579));
#64034=CARTESIAN_POINT('Ctrl Pts',(-6.14174450682077,3.82192100742865,-20.4481152762486));
#64035=CARTESIAN_POINT('Ctrl Pts',(-6.23193279862032,3.57829312430292,-20.1221434396294));
#64036=CARTESIAN_POINT('Ctrl Pts',(-6.16282464935142,3.57824724809887,-20.1925063319507));
#64037=CARTESIAN_POINT('Ctrl Pts',(-6.09371017736473,3.5782021591493,-20.2628625060442));
#64038=CARTESIAN_POINT('Ctrl Pts',(-6.02458951791509,3.57815724852431,-20.3332121247398));
#64039=CARTESIAN_POINT('Ctrl Pts',(-6.08725162051385,3.5,-19.9803008039646));
#64040=CARTESIAN_POINT('Ctrl Pts',(-6.01819267947756,3.50000086638443,-20.0506924537051));
#64041=CARTESIAN_POINT('Ctrl Pts',(-5.94912751219404,3.49999915309729,-20.121077743867));
#64042=CARTESIAN_POINT('Ctrl Pts',(-5.88005496058487,3.5,-20.1914556678078));
#64043=CARTESIAN_POINT('Ctrl Pts',(-6.,3.5,-19.8947609985686));
#64044=CARTESIAN_POINT('Ctrl Pts',(-5.93097159104175,3.5,-19.9651707980205));
#64045=CARTESIAN_POINT('Ctrl Pts',(-5.86193592281863,3.5,-20.035573480735));
#64046=CARTESIAN_POINT('Ctrl Pts',(-5.79289321881345,3.5,-20.1059692628831));
#64047=CARTESIAN_POINT('Ctrl Pts',(-5.79289321881345,3.5,-20.1059692628831));
#64048=CARTESIAN_POINT('Ctrl Pts',(-5.86193592281863,3.5,-20.035573480735));
#64049=CARTESIAN_POINT('Ctrl Pts',(-5.93097159104175,3.5,-19.9651707980205));
#64050=CARTESIAN_POINT('Ctrl Pts',(-6.,3.5,-19.8947609985686));
#64051=CARTESIAN_POINT('Ctrl Pts',(-6.35355339059328,4.0696900903742,-20.2413779215594));
#64052=CARTESIAN_POINT('Ctrl Pts',(-6.28452498163503,4.06945303220773,-20.311835383442));
#64053=CARTESIAN_POINT('Ctrl Pts',(-6.2154893134119,4.06921836801198,-20.3822849943144));
#64054=CARTESIAN_POINT('Ctrl Pts',(-6.14644660940672,4.06898602743283,-20.4527269996663));
#64055=CARTESIAN_POINT('Origin',(11.6,4.,-20.1059692628831));
#64056=CARTESIAN_POINT('',(-2.5,3.50845720475183,-20.1975426238546));
#64057=CARTESIAN_POINT('Ctrl Pts',(-2.,4.09756097560975,-20.5963587570998));
#64058=CARTESIAN_POINT('Ctrl Pts',(-2.00101528119204,4.09655313881206,-20.596559262091));
#64059=CARTESIAN_POINT('Ctrl Pts',(-2.00203056456928,4.09554468173501,-20.5967566605907));
#64060=CARTESIAN_POINT('Ctrl Pts',(-2.05580187973614,4.0421021986728,-20.6070466944938));
#64061=CARTESIAN_POINT('Ctrl Pts',(-2.10884374679379,3.98771778608941,-20.6088074165326));
#64062=CARTESIAN_POINT('Ctrl Pts',(-2.20924193430949,3.88147391652575,-20.5945414427224));
#64063=CARTESIAN_POINT('Ctrl Pts',(-2.25735953173246,3.82895180434594,-20.579160995088));
#64064=CARTESIAN_POINT('Ctrl Pts',(-2.34609881089932,3.728199733546,-20.529374025357));
#64065=CARTESIAN_POINT('Ctrl Pts',(-2.38730845067544,3.67931541228552,-20.4946845355157));
#64066=CARTESIAN_POINT('Ctrl Pts',(-2.44629528850599,3.60381971113444,-20.414637889374));
#64067=CARTESIAN_POINT('Ctrl Pts',(-2.46720605754511,3.57485564306978,-20.3741519147674));
#64068=CARTESIAN_POINT('Ctrl Pts',(-2.49343634644932,3.53186471227267,-20.2873343735479));
#64069=CARTESIAN_POINT('Ctrl Pts',(-2.5,3.51702916902183,-20.2435547744773));
#64070=CARTESIAN_POINT('Ctrl Pts',(-2.5,3.50845720475183,-20.1975426238546));
#64071=CARTESIAN_POINT('',(-2.5,3.5,-20.1059692628831));
#64072=CARTESIAN_POINT('Origin',(-2.5,4.,-20.1059692628831));
#64073=CARTESIAN_POINT('',(11.6,3.5,-20.1059692628831));
#64074=CARTESIAN_POINT('Origin',(11.6,20.1059692628831,-4.));
#64075=CARTESIAN_POINT('',(11.6,20.1059692628831,-3.5));
#64076=CARTESIAN_POINT('Origin',(-6.5,18.,-3.5));
#64077=CARTESIAN_POINT('',(-6.,18.5741756210067,-3.5));
#64078=CARTESIAN_POINT('',(-6.,19.25,-3.5));
#64079=CARTESIAN_POINT('',(-2.49011275851364,18.5741756287074,-3.5));
#64080=CARTESIAN_POINT('',(5.75,18.5741756210067,-3.5));
#64081=CARTESIAN_POINT('Ctrl Pts',(-2.49011275851347,18.5741756287065,-3.5));
#64082=CARTESIAN_POINT('Ctrl Pts',(-2.49686768056593,18.6082253077097,-3.5));
#64083=CARTESIAN_POINT('Ctrl Pts',(-2.5,18.6430188324712,-3.5));
#64084=CARTESIAN_POINT('Ctrl Pts',(-2.5,18.6748493969831,-3.5));
#64085=CARTESIAN_POINT('Origin',(-6.,19.25,-4.));
#64086=CARTESIAN_POINT('',(-6.5,18.5741756210067,-4.));
#64087=CARTESIAN_POINT('',(-6.5,19.25,-4.));
#64088=CARTESIAN_POINT('Origin',(-6.,18.5741756210067,-4.));
#64089=CARTESIAN_POINT('Origin',(-2.,0.,0.));
#64090=CARTESIAN_POINT('',(-2.5,-20.1975426238546,-3.50845720475183));
#64091=CARTESIAN_POINT('Origin',(-2.5,0.,0.));
#64092=CARTESIAN_POINT('Ctrl Pts',(-2.,-20.5963587570998,-4.09756097560975));
#64093=CARTESIAN_POINT('Ctrl Pts',(-2.00101528119129,-20.5965592620909,
-4.0965531388128));
#64094=CARTESIAN_POINT('Ctrl Pts',(-2.00203056456968,-20.5967566605904,
-4.09554468173651));
#64095=CARTESIAN_POINT('Ctrl Pts',(-2.05580187972316,-20.607046694496,-4.04210219866254));
#64096=CARTESIAN_POINT('Ctrl Pts',(-2.10884374679332,-20.6088074165326,
-3.98771778608992));
#64097=CARTESIAN_POINT('Ctrl Pts',(-2.20924193430925,-20.5945414427225,
-3.88147391652601));
#64098=CARTESIAN_POINT('Ctrl Pts',(-2.25735953173235,-20.5791609950881,
-3.82895180434606));
#64099=CARTESIAN_POINT('Ctrl Pts',(-2.34609881089934,-20.529374025357,-3.72819973354597));
#64100=CARTESIAN_POINT('Ctrl Pts',(-2.38730845067544,-20.4946845355157,
-3.67931541228552));
#64101=CARTESIAN_POINT('Ctrl Pts',(-2.44629528850598,-20.414637889374,-3.60381971113446));
#64102=CARTESIAN_POINT('Ctrl Pts',(-2.46720605754511,-20.3741519147674,
-3.57485564306979));
#64103=CARTESIAN_POINT('Ctrl Pts',(-2.49343634644932,-20.2873343735479,
-3.53186471227267));
#64104=CARTESIAN_POINT('Ctrl Pts',(-2.5,-20.2435547744773,-3.51702916902183));
#64105=CARTESIAN_POINT('Ctrl Pts',(-2.5,-20.1975426238547,-3.50845720475183));
#64106=CARTESIAN_POINT('Origin',(-2.5,-19.75,2.77555756156289E-15));
#64107=CARTESIAN_POINT('',(-2.5,-18.6748493969831,-3.5));
#64108=CARTESIAN_POINT('Origin',(-2.5,0.,0.));
#64109=CARTESIAN_POINT('',(-2.5,-20.1059692628831,-3.5));
#64110=CARTESIAN_POINT('',(-2.5,-21.5,-3.5));
#64111=CARTESIAN_POINT('Origin',(-2.5,-20.1059692628831,-3.99999999999999));
#64112=CARTESIAN_POINT('Origin',(-5.79289321881344,-4.,20.1059692628831));
#64113=CARTESIAN_POINT('Origin',(-5.79289321881344,-4.,20.1059692628831));
#64114=CARTESIAN_POINT('Origin',(-6.,-4.,18.5741756210067));
#64115=CARTESIAN_POINT('',(-6.,-3.89473684210526,18.0853815257171));
#64116=CARTESIAN_POINT('Origin',(-6.,-4.,18.5741756210067));
#64117=CARTESIAN_POINT('Origin',(-6.,-4.,18.5741756210067));
#64118=CARTESIAN_POINT('Origin',(5.75,-4.,18.5741756210067));
#64119=CARTESIAN_POINT('',(-2.49011275698595,-3.5,18.5741756210067));
#64120=CARTESIAN_POINT('',(5.75,-3.5,18.5741756210067));
#64121=CARTESIAN_POINT('',(-2.,-3.89473684210526,18.0853815257171));
#64122=CARTESIAN_POINT('Ctrl Pts',(-2.49011275698595,-3.5,18.5741756210067));
#64123=CARTESIAN_POINT('Ctrl Pts',(-2.48031734397251,-3.5,18.5247996785933));
#64124=CARTESIAN_POINT('Ctrl Pts',(-2.46374257315005,-3.50729593903647,
18.4776012558686));
#64125=CARTESIAN_POINT('Ctrl Pts',(-2.41476836802978,-3.53660915976364,
18.3774000478142));
#64126=CARTESIAN_POINT('Ctrl Pts',(-2.3796567831271,-3.56195342180394,18.3274816176557));
#64127=CARTESIAN_POINT('Ctrl Pts',(-2.29338459766338,-3.62956958867484,
18.232217901755));
#64128=CARTESIAN_POINT('Ctrl Pts',(-2.23978806301794,-3.67485926714063,
18.1898427129628));
#64129=CARTESIAN_POINT('Ctrl Pts',(-2.12593686398508,-3.77570829974231,
18.122961239244));
#64130=CARTESIAN_POINT('Ctrl Pts',(-2.06428277651074,-3.83280835545914,
18.0991128412042));
#64131=CARTESIAN_POINT('Ctrl Pts',(-2.00210742973619,-3.89270461507943,
18.0858224890517));
#64132=CARTESIAN_POINT('Ctrl Pts',(-2.00105371344565,-3.89372038856671,
18.0856004217928));
#64133=CARTESIAN_POINT('Ctrl Pts',(-2.,-3.89473684210526,18.0853815257171));
#64134=CARTESIAN_POINT('',(5.75,-3.89473684210526,18.0853815257171));
#64135=CARTESIAN_POINT('Origin',(-6.5,-3.5,21.5));
#64136=CARTESIAN_POINT('',(-2.5,-3.5,20.1059692628831));
#64137=CARTESIAN_POINT('',(11.6,-3.5,20.1059692628831));
#64138=CARTESIAN_POINT('',(-2.5,-3.5,18.6748493969831));
#64139=CARTESIAN_POINT('',(-2.5,-3.5,21.5));
#64140=CARTESIAN_POINT('Ctrl Pts',(-2.49011275698578,-3.5,18.5741756210058));
#64141=CARTESIAN_POINT('Ctrl Pts',(-2.49686768006346,-3.5,18.608225302467));
#64142=CARTESIAN_POINT('Ctrl Pts',(-2.5,-3.5,18.643018830074));
#64143=CARTESIAN_POINT('Ctrl Pts',(-2.5,-3.5,18.6748493969831));
#64144=CARTESIAN_POINT('Origin',(11.6,-4.,20.1059692628831));
#64145=CARTESIAN_POINT('',(-2.5,-3.50845720475185,20.1975426238546));
#64146=CARTESIAN_POINT('Ctrl Pts',(-2.,-4.09756097560976,20.5963587570998));
#64147=CARTESIAN_POINT('Ctrl Pts',(-2.00105378229977,-4.09651492000783,
20.5965668655651));
#64148=CARTESIAN_POINT('Ctrl Pts',(-2.00210756704266,-4.0954681961015,20.5967716274829));
#64149=CARTESIAN_POINT('Ctrl Pts',(-2.0549061979377,-4.04299001366594,20.6068632667935));
#64150=CARTESIAN_POINT('Ctrl Pts',(-2.10691928575593,-3.98968902087216,
20.6087335302367));
#64151=CARTESIAN_POINT('Ctrl Pts',(-2.20527868202034,-3.88572666709869,
20.5954171359809));
#64152=CARTESIAN_POINT('Ctrl Pts',(-2.25234932765368,-3.83445109616703,
20.5809320554912));
#64153=CARTESIAN_POINT('Ctrl Pts',(-2.34137513158209,-3.73373520421152,
20.5329716863835));
#64154=CARTESIAN_POINT('Ctrl Pts',(-2.38366457683681,-3.68376379464004,
20.4984471810012));
#64155=CARTESIAN_POINT('Ctrl Pts',(-2.44417869145193,-3.60667572573032,
20.4183174732899));
#64156=CARTESIAN_POINT('Ctrl Pts',(-2.46565574270481,-3.57712046761784,
20.377790317302));
#64157=CARTESIAN_POINT('Ctrl Pts',(-2.49271418520348,-3.53326962999165,
20.2909211660461));
#64158=CARTESIAN_POINT('Ctrl Pts',(-2.49963949791362,-3.5180773748747,20.2472123458134));
#64159=CARTESIAN_POINT('Ctrl Pts',(-2.49999544513914,-3.5089131932808,20.1999653820114));
#64160=CARTESIAN_POINT('Ctrl Pts',(-2.5,-3.50868289295355,20.1987540614206));
#64161=CARTESIAN_POINT('Ctrl Pts',(-2.5,-3.50845720475181,20.1975426238545));
#64162=CARTESIAN_POINT('Origin',(-2.5,-4.,20.1059692628831));
#64163=CARTESIAN_POINT('Origin',(-6.,4.,19.8947609985686));
#64164=CARTESIAN_POINT('',(-6.,3.5,19.8947609985686));
#64165=CARTESIAN_POINT('Origin',(-6.,4.,19.8947609985686));
#64166=CARTESIAN_POINT('Origin',(-6.,4.,19.8947609985686));
#64167=CARTESIAN_POINT('Ctrl Pts',(-6.,3.5,19.8947609985686));
#64168=CARTESIAN_POINT('Ctrl Pts',(-5.93097160224944,3.5,19.9651707865886));
#64169=CARTESIAN_POINT('Ctrl Pts',(-5.86193594526217,3.5,20.0355734578471));
#64170=CARTESIAN_POINT('Ctrl Pts',(-5.79289325246939,3.5,20.1059692285676));
#64171=CARTESIAN_POINT('Ctrl Pts',(-6.05816774700923,3.5,19.9517875354993));
#64172=CARTESIAN_POINT('Ctrl Pts',(-5.98911911240786,3.50000009695086,20.0221853297161));
#64173=CARTESIAN_POINT('Ctrl Pts',(-5.92006355655825,3.4999999051411,20.0925761964034));
#64174=CARTESIAN_POINT('Ctrl Pts',(-5.85100108032663,3.5,20.1629601651898));
#64175=CARTESIAN_POINT('Ctrl Pts',(-6.17423130798436,3.54067994796936,20.0655740114515));
#64176=CARTESIAN_POINT('Ctrl Pts',(-6.10514246533496,3.54065679708597,20.1359480490754));
#64177=CARTESIAN_POINT('Ctrl Pts',(-6.03604762835117,3.54063392422494,20.2063157629463));
#64178=CARTESIAN_POINT('Ctrl Pts',(-5.96694584478107,3.54061125868084,20.2766763539781));
#64179=CARTESIAN_POINT('Ctrl Pts',(-6.33051862687158,3.7371471217482,20.218795083619));
#64180=CARTESIAN_POINT('Ctrl Pts',(-6.26140158434861,3.73702083789835,20.2891625165557));
#64181=CARTESIAN_POINT('Ctrl Pts',(-6.19227810058116,3.73689571001199,20.3595229318531));
#64182=CARTESIAN_POINT('Ctrl Pts',(-6.12314873716634,3.73677204608588,20.4298768687522));
#64183=CARTESIAN_POINT('Ctrl Pts',(-6.36571453723109,3.94869478956009,20.2533004750967));
#64184=CARTESIAN_POINT('Ctrl Pts',(-6.29663983008132,3.94848324316203,20.3237142415202));
#64185=CARTESIAN_POINT('Ctrl Pts',(-6.22756051190152,3.94827447000558,20.3941224802241));
#64186=CARTESIAN_POINT('Ctrl Pts',(-6.15847252770227,3.94806722427235,20.4645217002994));
#64187=CARTESIAN_POINT('Ctrl Pts',(-6.35355339059327,4.0696900903742,20.2413779215594));
#64188=CARTESIAN_POINT('Ctrl Pts',(-6.28452499284272,4.06945303224623,20.3118353720023));
#64189=CARTESIAN_POINT('Ctrl Pts',(-6.21548933585545,4.06921836808827,20.3822849714111));
#64190=CARTESIAN_POINT('Ctrl Pts',(-6.14644664306266,4.06898602754609,20.4527269653283));
#64191=CARTESIAN_POINT('',(-5.79289325247318,3.5,20.1059692285637));
#64192=CARTESIAN_POINT('Origin',(-5.79289325247318,4.,20.1059692285637));
#64193=CARTESIAN_POINT('Ctrl Pts',(-6.,3.5,19.8947609985686));
#64194=CARTESIAN_POINT('Ctrl Pts',(-5.93097160224944,3.5,19.9651707865886));
#64195=CARTESIAN_POINT('Ctrl Pts',(-5.86193594526217,3.5,20.0355734578471));
#64196=CARTESIAN_POINT('Ctrl Pts',(-5.79289325246939,3.5,20.1059692285676));
#64197=CARTESIAN_POINT('Origin',(11.6,4.,20.1059692628831));
#64198=CARTESIAN_POINT('Origin',(-5.79289321881345,4.,20.1059692628831));
#64199=CARTESIAN_POINT('',(-2.5,3.5,20.1059692628831));
#64200=CARTESIAN_POINT('',(11.6,3.5,20.1059692628831));
#64201=CARTESIAN_POINT('',(-2.5,3.50845720475185,20.1975426238546));
#64202=CARTESIAN_POINT('Origin',(-2.5,4.,20.1059692628831));
#64203=CARTESIAN_POINT('Ctrl Pts',(-2.5,3.50845720475184,20.1975426238546));
#64204=CARTESIAN_POINT('Ctrl Pts',(-2.5,3.517036693927,20.2435951662777));
#64205=CARTESIAN_POINT('Ctrl Pts',(-2.49342483977402,3.53189060449051,20.287410477654));
#64206=CARTESIAN_POINT('Ctrl Pts',(-2.46710761937579,3.57500889896805,20.3744340358278));
#64207=CARTESIAN_POINT('Ctrl Pts',(-2.44607731612422,3.60411954186725,20.4150481564303));
#64208=CARTESIAN_POINT('Ctrl Pts',(-2.3866307647472,3.68015463370752,20.4954497474577));
#64209=CARTESIAN_POINT('Ctrl Pts',(-2.3450061363464,3.72948787520241,20.5302485483201));
#64210=CARTESIAN_POINT('Ctrl Pts',(-2.2561617458898,3.83026319150449,20.579566056646));
#64211=CARTESIAN_POINT('Ctrl Pts',(-2.20846377743015,3.88230470098185,20.5946909756454));
#64212=CARTESIAN_POINT('Ctrl Pts',(-2.10864661377827,3.98791865791761,20.608794231553));
#64213=CARTESIAN_POINT('Ctrl Pts',(-2.05576282506689,4.04213858560532,20.607026997786));
#64214=CARTESIAN_POINT('Ctrl Pts',(-2.00210756704338,4.09546819610263,20.5967716274827));
#64215=CARTESIAN_POINT('Ctrl Pts',(-2.00105378229923,4.09651492000836,20.596566865565));
#64216=CARTESIAN_POINT('Ctrl Pts',(-2.,4.09756097560976,20.5963587570998));
#64217=CARTESIAN_POINT('Origin',(-2.,0.,0.));
#64218=CARTESIAN_POINT('Origin',(-2.5,0.,0.));
#64219=CARTESIAN_POINT('Origin',(-5.79289321881345,4.,20.1059692628831));
#64220=CARTESIAN_POINT('Origin',(-6.5,3.5,18.));
#64221=CARTESIAN_POINT('',(-6.,3.5,18.5741756210067));
#64222=CARTESIAN_POINT('',(-6.,3.5,9.));
#64223=CARTESIAN_POINT('',(-2.49011275698595,3.5,18.5741756210067));
#64224=CARTESIAN_POINT('',(5.75,3.5,18.5741756210067));
#64225=CARTESIAN_POINT('',(-2.5,3.5,18.6748493969831));
#64226=CARTESIAN_POINT('Ctrl Pts',(-2.5,3.5,18.6748493969831));
#64227=CARTESIAN_POINT('Ctrl Pts',(-2.5,3.5,18.643018830074));
#64228=CARTESIAN_POINT('Ctrl Pts',(-2.49686768006346,3.5,18.608225302467));
#64229=CARTESIAN_POINT('Ctrl Pts',(-2.49011275698578,3.5,18.5741756210058));
#64230=CARTESIAN_POINT('',(-2.5,3.5,18.));
#64231=CARTESIAN_POINT('Origin',(-6.,4.,9.));
#64232=CARTESIAN_POINT('',(-6.5,4.,18.5741756210067));
#64233=CARTESIAN_POINT('',(-6.5,4.,9.));
#64234=CARTESIAN_POINT('Origin',(-6.,4.,18.5741756210067));
#64235=CARTESIAN_POINT('Origin',(-6.5,20.5,0.));
#64236=CARTESIAN_POINT('',(-6.5,18.5741756210067,4.));
#64237=CARTESIAN_POINT('',(-6.5,21.,4.));
#64238=CARTESIAN_POINT('Origin',(-6.5,0.,0.));
#64239=CARTESIAN_POINT('Origin',(-6.,21.,4.));
#64240=CARTESIAN_POINT('',(-6.,18.5741756210067,3.5));
#64241=CARTESIAN_POINT('',(-6.,21.,3.5));
#64242=CARTESIAN_POINT('Origin',(-6.,18.5741756210067,4.));
#64243=CARTESIAN_POINT('Origin',(-6.,18.5741756210067,4.));
#64244=CARTESIAN_POINT('',(-6.,18.0853815257171,3.89473684210526));
#64245=CARTESIAN_POINT('Origin',(-6.,18.5741756210067,4.));
#64246=CARTESIAN_POINT('Origin',(-6.,18.5741756210067,4.));
#64247=CARTESIAN_POINT('Origin',(-2.,0.,0.));
#64248=CARTESIAN_POINT('',(-2.5,-3.50845720475184,-20.1975426238546));
#64249=CARTESIAN_POINT('Ctrl Pts',(-2.5,-3.50845720475184,-20.1975426238546));
#64250=CARTESIAN_POINT('Ctrl Pts',(-2.5,-3.51702916902184,-20.2435547744772));
#64251=CARTESIAN_POINT('Ctrl Pts',(-2.49343634644932,-3.53186471227267,
-20.2873343735479));
#64252=CARTESIAN_POINT('Ctrl Pts',(-2.46720605754511,-3.57485564306979,
-20.3741519147674));
#64253=CARTESIAN_POINT('Ctrl Pts',(-2.44629528850598,-3.60381971113447,
-20.414637889374));
#64254=CARTESIAN_POINT('Ctrl Pts',(-2.38730845067544,-3.67931541228553,
-20.4946845355157));
#64255=CARTESIAN_POINT('Ctrl Pts',(-2.34609881089932,-3.72819973354599,
-20.529374025357));
#64256=CARTESIAN_POINT('Ctrl Pts',(-2.25735953173236,-3.82895180434606,
-20.5791609950881));
#64257=CARTESIAN_POINT('Ctrl Pts',(-2.20924193430928,-3.88147391652601,
-20.5945414427225));
#64258=CARTESIAN_POINT('Ctrl Pts',(-2.10884374679334,-3.98771778608992,
-20.6088074165326));
#64259=CARTESIAN_POINT('Ctrl Pts',(-2.05580187972934,-4.04210219866796,
-20.6070466944948));
#64260=CARTESIAN_POINT('Ctrl Pts',(-2.00203056456934,-4.09554468173591,
-20.5967566605905));
#64261=CARTESIAN_POINT('Ctrl Pts',(-2.00101528119147,-4.09655313881263,
-20.5965592620909));
#64262=CARTESIAN_POINT('Ctrl Pts',(-2.,-4.09756097560976,-20.5963587570998));
#64263=CARTESIAN_POINT('Origin',(-2.5,0.,0.));
#64264=CARTESIAN_POINT('Origin',(-2.5,-3.33066907387547E-15,-19.75));
#64265=CARTESIAN_POINT('',(-2.5,-3.5,-20.1059692628831));
#64266=CARTESIAN_POINT('Origin',(-2.5,-4.,-20.1059692628831));
#64267=CARTESIAN_POINT('',(-2.5,-3.5,-18.6748493969831));
#64268=CARTESIAN_POINT('',(-2.5,-3.5,-18.));
#64269=CARTESIAN_POINT('',(-2.5,3.5,-18.6748493969831));
#64270=CARTESIAN_POINT('Origin',(-2.5,0.,0.));
#64271=CARTESIAN_POINT('',(-2.5,3.5,-21.5));
#64272=CARTESIAN_POINT('Origin',(-2.,0.,0.));
#64273=CARTESIAN_POINT('',(-2.,-3.89473684210527,-18.0853815257171));
#64274=CARTESIAN_POINT('',(-2.49011275851364,-3.5,-18.5741756287074));
#64275=CARTESIAN_POINT('Ctrl Pts',(-2.,-3.89473684210527,-18.0853815257171));
#64276=CARTESIAN_POINT('Ctrl Pts',(-2.00094797695669,-3.89382238615325,
-18.085578456331));
#64277=CARTESIAN_POINT('Ctrl Pts',(-2.00189595598416,-3.89290848084184,
-18.0857779535775));
#64278=CARTESIAN_POINT('Ctrl Pts',(-2.09304035837669,-3.80509320931406,
-18.105205568777));
#64279=CARTESIAN_POINT('Ctrl Pts',(-2.18153986698468,-3.7247983724995,-18.1472832140884));
#64280=CARTESIAN_POINT('Ctrl Pts',(-2.3185279168613,-3.60890246257771,-18.2551075840637));
#64281=CARTESIAN_POINT('Ctrl Pts',(-2.3696986038289,-3.56883721926646,-18.3118008095372));
#64282=CARTESIAN_POINT('Ctrl Pts',(-2.43934686237775,-3.52083652884264,
-18.4222997616512));
#64283=CARTESIAN_POINT('Ctrl Pts',(-2.46399052835428,-3.50656062686055,
-18.4752127841392));
#64284=CARTESIAN_POINT('Ctrl Pts',(-2.48396330014831,-3.50059284622875,
-18.54612986876));
#64285=CARTESIAN_POINT('Ctrl Pts',(-2.48732407582936,-3.49999999978351,
-18.560118656735));
#64286=CARTESIAN_POINT('Ctrl Pts',(-2.49011275851364,-3.5,-18.5741756287074));
#64287=CARTESIAN_POINT('',(-2.,3.89473684210526,-18.0853815257171));
#64288=CARTESIAN_POINT('Origin',(-2.,0.,0.));
#64289=CARTESIAN_POINT('',(-2.49011275851364,3.5,-18.5741756287073));
#64290=CARTESIAN_POINT('Ctrl Pts',(-2.49011275851364,3.5,-18.5741756287073));
#64291=CARTESIAN_POINT('Ctrl Pts',(-2.48732407582936,3.4999999997835,-18.560118656735));
#64292=CARTESIAN_POINT('Ctrl Pts',(-2.48396330014829,3.50059284622874,-18.5461298687599));
#64293=CARTESIAN_POINT('Ctrl Pts',(-2.46399052835424,3.50656062686056,-18.4752127841391));
#64294=CARTESIAN_POINT('Ctrl Pts',(-2.4393468623777,3.52083652884266,-18.4222997616511));
#64295=CARTESIAN_POINT('Ctrl Pts',(-2.36969860382856,3.5688372192667,-18.3118008095367));
#64296=CARTESIAN_POINT('Ctrl Pts',(-2.31852791686079,3.60890246257814,-18.2551075840632));
#64297=CARTESIAN_POINT('Ctrl Pts',(-2.1815398669833,3.72479837250067,-18.1472832140873));
#64298=CARTESIAN_POINT('Ctrl Pts',(-2.09304035837488,3.80509320931587,-18.1052055687765));
#64299=CARTESIAN_POINT('Ctrl Pts',(-2.00189595598381,3.89290848084216,-18.0857779535774));
#64300=CARTESIAN_POINT('Ctrl Pts',(-2.0009479769565,3.89382238615342,-18.0855784563309));
#64301=CARTESIAN_POINT('Ctrl Pts',(-2.,3.89473684210526,-18.0853815257171));
#64302=CARTESIAN_POINT('Ctrl Pts',(-2.5,3.5,-18.6748493969831));
#64303=CARTESIAN_POINT('Ctrl Pts',(-2.5,3.5,-18.6430188324712));
#64304=CARTESIAN_POINT('Ctrl Pts',(-2.49686768056593,3.5,-18.6082253077096));
#64305=CARTESIAN_POINT('Ctrl Pts',(-2.49011275851347,3.5,-18.5741756287065));
#64306=CARTESIAN_POINT('Ctrl Pts',(-2.49011275851347,-3.5,-18.5741756287065));
#64307=CARTESIAN_POINT('Ctrl Pts',(-2.49686768056593,-3.5,-18.6082253077096));
#64308=CARTESIAN_POINT('Ctrl Pts',(-2.5,-3.5,-18.6430188324712));
#64309=CARTESIAN_POINT('Ctrl Pts',(-2.5,-3.5,-18.6748493969831));
#64310=CARTESIAN_POINT('Origin',(-6.,0.,0.));
#64311=CARTESIAN_POINT('',(-6.,3.89473684210526,18.0853815257171));
#64312=CARTESIAN_POINT('Origin',(-6.,0.,0.));
#64313=CARTESIAN_POINT('Origin',(-6.,4.,18.5741756210067));
#64314=CARTESIAN_POINT('Origin',(5.75,18.5741756210067,4.));
#64315=CARTESIAN_POINT('',(-2.49011275698595,18.5741756210067,3.5));
#64316=CARTESIAN_POINT('',(5.75,18.5741756210067,3.5));
#64317=CARTESIAN_POINT('',(-2.,18.0853815257171,3.89473684210526));
#64318=CARTESIAN_POINT('Ctrl Pts',(-2.49011275698595,18.5741756210067,3.5));
#64319=CARTESIAN_POINT('Ctrl Pts',(-2.4803173439725,18.5247996785932,3.5));
#64320=CARTESIAN_POINT('Ctrl Pts',(-2.46374257315002,18.4776012558685,3.5072959390365));
#64321=CARTESIAN_POINT('Ctrl Pts',(-2.41476836802979,18.3774000478142,3.53660915976365));
#64322=CARTESIAN_POINT('Ctrl Pts',(-2.37965678312714,18.3274816176558,3.5619534218039));
#64323=CARTESIAN_POINT('Ctrl Pts',(-2.29338459766337,18.232217901755,3.62956958867484));
#64324=CARTESIAN_POINT('Ctrl Pts',(-2.23978806301794,18.1898427129628,3.67485926714064));
#64325=CARTESIAN_POINT('Ctrl Pts',(-2.12593686398496,18.1229612392439,3.77570829974241));
#64326=CARTESIAN_POINT('Ctrl Pts',(-2.0642827765073,18.0991128412049,3.83280835545585));
#64327=CARTESIAN_POINT('Ctrl Pts',(-2.00210742973639,18.0858224890517,3.89270461507972));
#64328=CARTESIAN_POINT('Ctrl Pts',(-2.00105371344551,18.0856004217928,3.89372038856684));
#64329=CARTESIAN_POINT('Ctrl Pts',(-2.,18.0853815257171,3.89473684210526));
#64330=CARTESIAN_POINT('',(5.75,18.0853815257171,3.89473684210526));
#64331=CARTESIAN_POINT('Origin',(-2.,0.,0.));
#64332=CARTESIAN_POINT('',(-2.,18.0853815257171,-3.89473684210526));
#64333=CARTESIAN_POINT('Ctrl Pts',(-2.,18.0853815257171,-3.89473684210527));
#64334=CARTESIAN_POINT('Ctrl Pts',(-2.00094797695641,18.0855784563309,-3.89382238615351));
#64335=CARTESIAN_POINT('Ctrl Pts',(-2.00189595598414,18.0857779535775,-3.89290848084185));
#64336=CARTESIAN_POINT('Ctrl Pts',(-2.09304035837568,18.1052055687767,-3.80509320931504));
#64337=CARTESIAN_POINT('Ctrl Pts',(-2.1815398669839,18.1472832140878,-3.72479837250016));
#64338=CARTESIAN_POINT('Ctrl Pts',(-2.31852791686109,18.2551075840635,-3.60890246257788));
#64339=CARTESIAN_POINT('Ctrl Pts',(-2.36969860382876,18.311800809537,-3.56883721926657));
#64340=CARTESIAN_POINT('Ctrl Pts',(-2.43934686237771,18.4222997616511,-3.52083652884266));
#64341=CARTESIAN_POINT('Ctrl Pts',(-2.46399052835424,18.4752127841391,-3.50656062686056));
#64342=CARTESIAN_POINT('Ctrl Pts',(-2.48396330014829,18.5461298687599,-3.50059284622875));
#64343=CARTESIAN_POINT('Ctrl Pts',(-2.48732407582936,18.560118656735,-3.4999999997835));
#64344=CARTESIAN_POINT('Ctrl Pts',(-2.49011275851364,18.5741756287074,-3.5));
#64345=CARTESIAN_POINT('Origin',(-2.,0.,0.));
#64346=CARTESIAN_POINT('Ctrl Pts',(-2.49011275698578,18.5741756210058,3.5));
#64347=CARTESIAN_POINT('Ctrl Pts',(-2.49686768006346,18.608225302467,3.5));
#64348=CARTESIAN_POINT('Ctrl Pts',(-2.5,18.643018830074,3.5));
#64349=CARTESIAN_POINT('Ctrl Pts',(-2.5,18.6748493969831,3.5));
#64350=CARTESIAN_POINT('Origin',(-6.,4.,18.5741756210067));
#64351=CARTESIAN_POINT('Origin',(-6.,4.,18.5741756210067));
#64352=CARTESIAN_POINT('Origin',(5.75,4.,18.5741756210067));
#64353=CARTESIAN_POINT('',(-2.,3.89473684210526,18.0853815257171));
#64354=CARTESIAN_POINT('',(5.75,3.89473684210526,18.0853815257171));
#64355=CARTESIAN_POINT('Ctrl Pts',(-2.,3.89473684210526,18.0853815257171));
#64356=CARTESIAN_POINT('Ctrl Pts',(-2.00105371344572,3.89372038856664,18.0856004217929));
#64357=CARTESIAN_POINT('Ctrl Pts',(-2.00210742973654,3.89270461507958,18.0858224890517));
#64358=CARTESIAN_POINT('Ctrl Pts',(-2.09351569465547,3.804646993342,18.1053615522589));
#64359=CARTESIAN_POINT('Ctrl Pts',(-2.18214848766776,3.72425195645496,18.1476027839865));
#64360=CARTESIAN_POINT('Ctrl Pts',(-2.31958013153081,3.60803698471264,18.2560609577767));
#64361=CARTESIAN_POINT('Ctrl Pts',(-2.37098023972695,3.56784861835865,18.3132986190986));
#64362=CARTESIAN_POINT('Ctrl Pts',(-2.44048867507143,3.52013110417152,18.4245257150294));
#64363=CARTESIAN_POINT('Ctrl Pts',(-2.46491477585542,3.50609467152981,18.4775461366035));
#64364=CARTESIAN_POINT('Ctrl Pts',(-2.48434736805698,3.50052662530646,18.5477361044576));
#64365=CARTESIAN_POINT('Ctrl Pts',(-2.48748442178262,3.5,18.5609269169995));
#64366=CARTESIAN_POINT('Ctrl Pts',(-2.49011275698595,3.5,18.5741756210067));
#64367=CARTESIAN_POINT('Origin',(5.75,0.,0.));
#64368=CARTESIAN_POINT('',(7.5,14.9828768864291,-10.8518846384445));
#64369=CARTESIAN_POINT('',(5.75,14.9828768864291,-10.8518846384445));
#64370=CARTESIAN_POINT('',(7.5,14.9828768864291,10.8518846384445));
#64371=CARTESIAN_POINT('',(5.75,14.9828768864291,10.8518846384445));
#64372=CARTESIAN_POINT('',(7.5,10.8518846384445,14.9828768864291));
#64373=CARTESIAN_POINT('Origin',(7.5,0.,0.));
#64374=CARTESIAN_POINT('',(5.75,10.8518846384445,14.9828768864291));
#64375=CARTESIAN_POINT('',(7.5,-10.8518846384445,14.9828768864291));
#64376=CARTESIAN_POINT('',(5.75,-10.8518846384445,14.9828768864291));
#64377=CARTESIAN_POINT('',(7.5,-14.9828768864291,10.8518846384445));
#64378=CARTESIAN_POINT('Origin',(7.5,0.,0.));
#64379=CARTESIAN_POINT('',(5.75,-14.9828768864291,10.8518846384445));
#64380=CARTESIAN_POINT('',(-2.,-18.5,-2.2655965784226E-15));
#64381=CARTESIAN_POINT('',(5.75,-18.5,-2.2655965784226E-15));
#64382=CARTESIAN_POINT('',(-2.,-18.0853815257171,3.89473684210527));
#64383=CARTESIAN_POINT('Origin',(-2.,0.,0.));
#64384=CARTESIAN_POINT('',(5.75,-18.0853815257171,3.89473684210527));
#64385=CARTESIAN_POINT('Origin',(-6.,0.,0.));
#64386=CARTESIAN_POINT('Origin',(-2.,0.,0.));
#64387=CARTESIAN_POINT('',(-6.,18.0853815257171,-3.89473684210526));
#64388=CARTESIAN_POINT('',(5.75,18.0853815257171,-3.89473684210526));
#64389=CARTESIAN_POINT('',(-6.,3.89473684210526,-18.0853815257171));
#64390=CARTESIAN_POINT('Origin',(-6.,0.,0.));
#64391=CARTESIAN_POINT('',(5.75,3.89473684210526,-18.0853815257171));
#64392=CARTESIAN_POINT('',(-6.,-3.89473684210527,-18.0853815257171));
#64393=CARTESIAN_POINT('',(5.75,-3.89473684210527,-18.0853815257171));
#64394=CARTESIAN_POINT('',(-6.,-18.0853815257171,-3.89473684210526));
#64395=CARTESIAN_POINT('Origin',(-6.,0.,0.));
#64396=CARTESIAN_POINT('',(-2.,-18.0853815257171,-3.89473684210526));
#64397=CARTESIAN_POINT('',(5.75,-18.0853815257171,-3.89473684210526));
#64398=CARTESIAN_POINT('Origin',(-2.,0.,0.));
#64399=CARTESIAN_POINT('',(7.5,-14.9828768864291,-10.8518846384445));
#64400=CARTESIAN_POINT('',(5.75,-14.9828768864291,-10.8518846384445));
#64401=CARTESIAN_POINT('',(7.5,-10.8518846384445,-14.9828768864291));
#64402=CARTESIAN_POINT('Origin',(7.5,0.,0.));
#64403=CARTESIAN_POINT('',(5.75,-10.8518846384445,-14.9828768864291));
#64404=CARTESIAN_POINT('',(7.5,10.8518846384445,-14.9828768864291));
#64405=CARTESIAN_POINT('',(5.75,10.8518846384445,-14.9828768864291));
#64406=CARTESIAN_POINT('Origin',(7.5,0.,0.));
#64407=CARTESIAN_POINT('Origin',(5.75,15.3878195049812,-11.145178817862));
#64408=CARTESIAN_POINT('',(7.99471483544825,15.034266114388,-11.4987322084552));
#64409=CARTESIAN_POINT('',(5.75,15.034266114388,-11.4987322084552));
#64410=CARTESIAN_POINT('Ctrl Pts',(7.5,14.9828768864291,-10.8518846384445));
#64411=CARTESIAN_POINT('Ctrl Pts',(7.50105371344594,14.9822669774522,-10.8527267217709));
#64412=CARTESIAN_POINT('Ctrl Pts',(7.50210742973669,14.9816596935127,-10.8535707098414));
#64413=CARTESIAN_POINT('Ctrl Pts',(7.59351569467899,14.9292065753492,-10.9269504763462));
#64414=CARTESIAN_POINT('Ctrl Pts',(7.68214848767697,14.8976245327992,-11.0120989243868));
#64415=CARTESIAN_POINT('Ctrl Pts',(7.81958013152899,14.8836434033438,-11.1704454530317));
#64416=CARTESIAN_POINT('Ctrl Pts',(7.87098023972546,14.8919941158644,-11.2398826207751));
#64417=CARTESIAN_POINT('Ctrl Pts',(7.94048867507039,14.9308215694372,-11.3545161973505));
#64418=CARTESIAN_POINT('Ctrl Pts',(7.96491477585465,14.9558097197837,-11.4033401554803));
#64419=CARTESIAN_POINT('Ctrl Pts',(7.98678347589511,15.0039319604954,-11.466290886942));
#64420=CARTESIAN_POINT('Ctrl Pts',(7.9914773312572,15.0185083904015,-11.4829744844688));
#64421=CARTESIAN_POINT('Ctrl Pts',(7.99471483544825,15.034266114388,-11.4987322084552));
#64422=CARTESIAN_POINT('Origin',(7.5,0.,0.));
#64423=CARTESIAN_POINT('',(7.99471483561597,11.4987322092715,-15.0342661152043));
#64424=CARTESIAN_POINT('Ctrl Pts',(7.99471483561596,11.4987322092715,-15.0342661152043));
#64425=CARTESIAN_POINT('Ctrl Pts',(7.9913625823211,11.4824159731374,-15.0179498789948));
#64426=CARTESIAN_POINT('Ctrl Pts',(7.98645003622193,11.4651126007102,-15.0029056934798));
#64427=CARTESIAN_POINT('Ctrl Pts',(7.96402271105306,11.4013638075407,-14.9546388364281));
#64428=CARTESIAN_POINT('Ctrl Pts',(7.93938632198296,11.3524620624659,-14.9298917928023));
#64429=CARTESIAN_POINT('Ctrl Pts',(7.86974221712864,11.2381679469927,-14.8917374982997));
#64430=CARTESIAN_POINT('Ctrl Pts',(7.81856316470143,11.1692008513045,-14.8836497863542));
#64431=CARTESIAN_POINT('Ctrl Pts',(7.68155929434285,11.0115152525768,-14.8978112789729));
#64432=CARTESIAN_POINT('Ctrl Pts',(7.59305526455752,10.9265492041506,-14.9294271056802));
#64433=CARTESIAN_POINT('Ctrl Pts',(7.50190235999067,10.8534064745166,-14.981777905381));
#64434=CARTESIAN_POINT('Ctrl Pts',(7.50095117894872,10.852644780527,-14.9823263263298));
#64435=CARTESIAN_POINT('Ctrl Pts',(7.5,10.8518846384445,-14.9828768864291));
#64436=CARTESIAN_POINT('',(8.,11.5504536489008,-15.0859875548336));
#64437=CARTESIAN_POINT('Ctrl Pts',(8.,11.5504536489008,-15.0859875548336));
#64438=CARTESIAN_POINT('Ctrl Pts',(8.,11.5339910291066,-15.0695249350393));
#64439=CARTESIAN_POINT('Ctrl Pts',(7.99834499880831,11.5164011008489,-15.0519350067816));
#64440=CARTESIAN_POINT('Ctrl Pts',(7.99471483561601,11.4987322092717,-15.0342661152045));
#64441=CARTESIAN_POINT('',(8.,15.0859875548336,-11.5504536489008));
#64442=CARTESIAN_POINT('Origin',(8.,0.,0.));
#64443=CARTESIAN_POINT('Ctrl Pts',(8.,15.0859875548336,-11.5504536489008));
#64444=CARTESIAN_POINT('Ctrl Pts',(8.,15.0695249347861,-11.5339910288533));
#64445=CARTESIAN_POINT('Ctrl Pts',(7.99834499875555,15.05193500624,-11.5164011003073));
#64446=CARTESIAN_POINT('Ctrl Pts',(7.9947148354483,15.0342661143882,-11.4987322084555));
#64447=CARTESIAN_POINT('Origin',(8.,13.3643181644257,-13.3643181644258));
#64448=CARTESIAN_POINT('',(8.,12.0208152801713,-15.556349186104));
#64449=CARTESIAN_POINT('',(8.,11.1722871427474,-14.7078210486802));
#64450=CARTESIAN_POINT('',(8.,15.556349186104,-12.0208152801713));
#64451=CARTESIAN_POINT('',(8.,12.0208152801713,-15.556349186104));
#64452=CARTESIAN_POINT('',(8.,15.556349186104,-12.0208152801713));
#64453=CARTESIAN_POINT('Origin',(5.75,-15.3878195049812,11.145178817862));
#64454=CARTESIAN_POINT('',(7.99471483544825,-15.034266114388,11.4987322084552));
#64455=CARTESIAN_POINT('',(5.75,-15.034266114388,11.4987322084552));
#64456=CARTESIAN_POINT('Ctrl Pts',(7.5,-14.9828768864291,10.8518846384445));
#64457=CARTESIAN_POINT('Ctrl Pts',(7.50105371344579,-14.9822669774523,10.8527267217707));
#64458=CARTESIAN_POINT('Ctrl Pts',(7.50210742973579,-14.9816596935132,10.8535707098407));
#64459=CARTESIAN_POINT('Ctrl Pts',(7.59351569467817,-14.9292065753492,10.9269504763458));
#64460=CARTESIAN_POINT('Ctrl Pts',(7.68214848767641,-14.8976245327994,11.0120989243863));
#64461=CARTESIAN_POINT('Ctrl Pts',(7.81958013152829,-14.8836434033437,11.1704454530308));
#64462=CARTESIAN_POINT('Ctrl Pts',(7.87098023972491,-14.8919941158642,11.2398826207743));
#64463=CARTESIAN_POINT('Ctrl Pts',(7.9404886750701,-14.9308215694369,11.3545161973499));
#64464=CARTESIAN_POINT('Ctrl Pts',(7.96491477585444,-14.9558097197834,11.4033401554798));
#64465=CARTESIAN_POINT('Ctrl Pts',(7.98678347589503,-15.0039319604951,11.4662908869417));
#64466=CARTESIAN_POINT('Ctrl Pts',(7.99147733125717,-15.0185083904014,11.4829744844687));
#64467=CARTESIAN_POINT('Ctrl Pts',(7.99471483544825,-15.034266114388,11.4987322084552));
#64468=CARTESIAN_POINT('Origin',(7.5,0.,0.));
#64469=CARTESIAN_POINT('',(7.99471483561596,-11.4987322092715,15.0342661152043));
#64470=CARTESIAN_POINT('Ctrl Pts',(7.99471483561596,-11.4987322092715,15.0342661152043));
#64471=CARTESIAN_POINT('Ctrl Pts',(7.99136258232109,-11.4824159731374,15.0179498789948));
#64472=CARTESIAN_POINT('Ctrl Pts',(7.98645003622191,-11.4651126007102,15.0029056934798));
#64473=CARTESIAN_POINT('Ctrl Pts',(7.964022711053,-11.4013638075406,14.954638836428));
#64474=CARTESIAN_POINT('Ctrl Pts',(7.93938632198288,-11.3524620624657,14.9298917928022));
#64475=CARTESIAN_POINT('Ctrl Pts',(7.86974221712845,-11.2381679469924,14.8917374982996));
#64476=CARTESIAN_POINT('Ctrl Pts',(7.81856316470117,-11.1692008513042,14.8836497863542));
#64477=CARTESIAN_POINT('Ctrl Pts',(7.68155929434292,-11.0115152525769,14.897811278973));
#64478=CARTESIAN_POINT('Ctrl Pts',(7.59305526455765,-10.9265492041507,14.9294271056801));
#64479=CARTESIAN_POINT('Ctrl Pts',(7.50190235999013,-10.8534064745162,14.9817779053813));
#64480=CARTESIAN_POINT('Ctrl Pts',(7.500951178949,-10.8526447805272,14.9823263263296));
#64481=CARTESIAN_POINT('Ctrl Pts',(7.5,-10.8518846384445,14.9828768864291));
#64482=CARTESIAN_POINT('',(8.,-11.5504536489008,15.0859875548336));
#64483=CARTESIAN_POINT('Ctrl Pts',(8.,-11.5504536489008,15.0859875548336));
#64484=CARTESIAN_POINT('Ctrl Pts',(8.,-11.5339910291066,15.0695249350393));
#64485=CARTESIAN_POINT('Ctrl Pts',(7.99834499880831,-11.5164011008489,15.0519350067816));
#64486=CARTESIAN_POINT('Ctrl Pts',(7.99471483561601,-11.4987322092717,15.0342661152045));
#64487=CARTESIAN_POINT('',(8.,-15.0859875548336,11.5504536489008));
#64488=CARTESIAN_POINT('Origin',(8.,0.,0.));
#64489=CARTESIAN_POINT('Ctrl Pts',(8.,-15.0859875548336,11.5504536489008));
#64490=CARTESIAN_POINT('Ctrl Pts',(8.,-15.0695249347861,11.5339910288533));
#64491=CARTESIAN_POINT('Ctrl Pts',(7.99834499875555,-15.05193500624,11.5164011003073));
#64492=CARTESIAN_POINT('Ctrl Pts',(7.9947148354483,-15.0342661143882,11.4987322084555));
#64493=CARTESIAN_POINT('Origin',(8.,-13.3643181644257,13.3643181644258));
#64494=CARTESIAN_POINT('',(8.,-12.0208152801713,15.556349186104));
#64495=CARTESIAN_POINT('',(8.,-11.1722871427475,14.7078210486802));
#64496=CARTESIAN_POINT('',(8.,-15.556349186104,12.0208152801713));
#64497=CARTESIAN_POINT('',(8.,-12.0208152801713,15.556349186104));
#64498=CARTESIAN_POINT('',(8.,-15.556349186104,12.0208152801713));
#64499=CARTESIAN_POINT('Origin',(5.75,-18.5741756210067,4.));
#64500=CARTESIAN_POINT('Ctrl Pts',(-2.,-18.0853815257171,3.89473684210527));
#64501=CARTESIAN_POINT('Ctrl Pts',(-2.00105371344577,-18.0856004217929,
3.89372038856659));
#64502=CARTESIAN_POINT('Ctrl Pts',(-2.00210742973639,-18.0858224890519,
3.8927046150788));
#64503=CARTESIAN_POINT('Ctrl Pts',(-2.09351569467844,-18.1053615522597,
3.80464699333924));
#64504=CARTESIAN_POINT('Ctrl Pts',(-2.1821484876768,-18.1476027839944,3.72425195644745));
#64505=CARTESIAN_POINT('Ctrl Pts',(-2.31958013152849,-18.2560609577744,
3.60803698471449));
#64506=CARTESIAN_POINT('Ctrl Pts',(-2.3709802397251,-18.3132986190962,3.56784861836004));
#64507=CARTESIAN_POINT('Ctrl Pts',(-2.44048867507028,-18.4245257150271,
3.52013110417223));
#64508=CARTESIAN_POINT('Ctrl Pts',(-2.46491477585457,-18.4775461366012,
3.50609467153023));
#64509=CARTESIAN_POINT('Ctrl Pts',(-2.48434736805665,-18.5477361044563,
3.50052662530652));
#64510=CARTESIAN_POINT('Ctrl Pts',(-2.48748442178248,-18.5609269169988,
3.5));
#64511=CARTESIAN_POINT('Ctrl Pts',(-2.49011275698595,-18.5741756210067,
3.5));
#64512=CARTESIAN_POINT('Origin',(-6.,0.,0.));
#64513=CARTESIAN_POINT('',(-6.5,-4.,-18.5741756210067));
#64514=CARTESIAN_POINT('Origin',(-6.,-4.00000000000001,-18.5741756210067));
#64515=CARTESIAN_POINT('',(-6.5,-18.6748493969831,-3.5));
#64516=CARTESIAN_POINT('Origin',(-6.5,0.,0.));
#64517=CARTESIAN_POINT('',(-6.49011275698595,-18.5741756210067,-3.5));
#64518=CARTESIAN_POINT('Ctrl Pts',(-6.5,-18.6748493969831,-3.5));
#64519=CARTESIAN_POINT('Ctrl Pts',(-6.5,-18.643018830074,-3.5));
#64520=CARTESIAN_POINT('Ctrl Pts',(-6.49686768006357,-18.6082253024678,
-3.5));
#64521=CARTESIAN_POINT('Ctrl Pts',(-6.49011275698595,-18.5741756210067,
-3.5));
#64522=CARTESIAN_POINT('Ctrl Pts',(-6.49011275698595,-18.5741756210067,
-3.5));
#64523=CARTESIAN_POINT('Ctrl Pts',(-6.48031734397251,-18.5247996785933,
-3.5));
#64524=CARTESIAN_POINT('Ctrl Pts',(-6.46374257315005,-18.4776012558686,
-3.50729593903647));
#64525=CARTESIAN_POINT('Ctrl Pts',(-6.41476836802977,-18.3774000478142,
-3.53660915976364));
#64526=CARTESIAN_POINT('Ctrl Pts',(-6.37965678312709,-18.3274816176557,
-3.56195342180394));
#64527=CARTESIAN_POINT('Ctrl Pts',(-6.29338459766337,-18.232217901755,-3.62956958867485));
#64528=CARTESIAN_POINT('Ctrl Pts',(-6.23978806301794,-18.1898427129628,
-3.67485926714064));
#64529=CARTESIAN_POINT('Ctrl Pts',(-6.12593686398507,-18.122961239244,-3.77570829974231));
#64530=CARTESIAN_POINT('Ctrl Pts',(-6.0642827765107,-18.0991128412042,-3.83280835545914));
#64531=CARTESIAN_POINT('Ctrl Pts',(-6.00210742973624,-18.0858224890518,
-3.89270461507938));
#64532=CARTESIAN_POINT('Ctrl Pts',(-6.0010537134456,-18.0856004217928,-3.89372038856676));
#64533=CARTESIAN_POINT('Ctrl Pts',(-6.,-18.0853815257171,-3.89473684210526));
#64534=CARTESIAN_POINT('Origin',(-6.,-4.,-18.5741756210067));
#64535=CARTESIAN_POINT('',(-6.,-3.5,-18.5741756210067));
#64536=CARTESIAN_POINT('Origin',(-6.,-4.,-18.5741756210067));
#64537=CARTESIAN_POINT('Origin',(-6.,-4.,-18.5741756210067));
#64538=CARTESIAN_POINT('Origin',(5.75,-18.5741756210067,-4.));
#64539=CARTESIAN_POINT('',(-2.49011275698595,-18.5741756210067,-3.5));
#64540=CARTESIAN_POINT('',(5.75,-18.5741756210067,-3.5));
#64541=CARTESIAN_POINT('Ctrl Pts',(-2.49011275698595,-18.5741756210067,
-3.5));
#64542=CARTESIAN_POINT('Ctrl Pts',(-2.48031734397251,-18.5247996785933,
-3.5));
#64543=CARTESIAN_POINT('Ctrl Pts',(-2.46374257315005,-18.4776012558686,
-3.50729593903647));
#64544=CARTESIAN_POINT('Ctrl Pts',(-2.41476836802978,-18.3774000478142,
-3.53660915976364));
#64545=CARTESIAN_POINT('Ctrl Pts',(-2.3796567831271,-18.3274816176557,-3.56195342180394));
#64546=CARTESIAN_POINT('Ctrl Pts',(-2.29338459766337,-18.232217901755,-3.62956958867485));
#64547=CARTESIAN_POINT('Ctrl Pts',(-2.23978806301794,-18.1898427129628,
-3.67485926714064));
#64548=CARTESIAN_POINT('Ctrl Pts',(-2.12593686398505,-18.122961239244,-3.77570829974233));
#64549=CARTESIAN_POINT('Ctrl Pts',(-2.06428277651057,-18.0991128412042,
-3.83280835545912));
#64550=CARTESIAN_POINT('Ctrl Pts',(-2.00210742973612,-18.0858224890517,
-3.89270461507951));
#64551=CARTESIAN_POINT('Ctrl Pts',(-2.0010537134457,-18.0856004217928,-3.89372038856666));
#64552=CARTESIAN_POINT('Ctrl Pts',(-2.,-18.0853815257171,-3.89473684210526));
#64553=CARTESIAN_POINT('Origin',(-2.,0.,0.));
#64554=CARTESIAN_POINT('Ctrl Pts',(-2.49011275698578,-18.5741756210058,
-3.5));
#64555=CARTESIAN_POINT('Ctrl Pts',(-2.49686768006346,-18.608225302467,-3.5));
#64556=CARTESIAN_POINT('Ctrl Pts',(-2.5,-18.643018830074,-3.5));
#64557=CARTESIAN_POINT('Ctrl Pts',(-2.5,-18.6748493969831,-3.5));
#64558=CARTESIAN_POINT('Origin',(-6.,0.,0.));
#64559=CARTESIAN_POINT('Origin',(-2.,0.,0.));
#64560=CARTESIAN_POINT('Origin',(-2.5,0.,0.));
#64561=CARTESIAN_POINT('Origin',(-2.5,1.11022302462516E-15,19.75));
#64562=CARTESIAN_POINT('Origin',(5.75,-4.,-18.5741756210067));
#64563=CARTESIAN_POINT('',(5.75,-3.5,-18.5741756210067));
#64564=CARTESIAN_POINT('Origin',(-6.,-4.,-9.));
#64565=CARTESIAN_POINT('',(-6.,-3.5,-20.1059692628831));
#64566=CARTESIAN_POINT('',(-6.,-3.5,-9.));
#64567=CARTESIAN_POINT('',(-6.5,-4.,-20.1059692628831));
#64568=CARTESIAN_POINT('Origin',(-6.,-4.,-20.1059692628831));
#64569=CARTESIAN_POINT('',(-6.5,-4.,-9.));
#64570=CARTESIAN_POINT('Origin',(-6.,-4.,-20.1059692628831));
#64571=CARTESIAN_POINT('Ctrl Pts',(-6.,-4.09756097560976,-20.5963587570998));
#64572=CARTESIAN_POINT('Ctrl Pts',(-6.,-4.0683589966744,-20.6021683708624));
#64573=CARTESIAN_POINT('Ctrl Pts',(-6.00276332358265,-4.03610462934205,
-20.6056974194132));
#64574=CARTESIAN_POINT('Ctrl Pts',(-6.01450725061641,-3.97271232495602,
-20.6060535888886));
#64575=CARTESIAN_POINT('Ctrl Pts',(-6.02348817950739,-3.94157444978542,
-20.6028809931646));
#64576=CARTESIAN_POINT('Ctrl Pts',(-6.04683850352093,-3.88079927444089,
-20.5906622808365));
#64577=CARTESIAN_POINT('Ctrl Pts',(-6.0663740221613,-3.84384286975754,-20.5777101026407));
#64578=CARTESIAN_POINT('Ctrl Pts',(-6.10731554914672,-3.78596404697746,
-20.5468117668285));
#64579=CARTESIAN_POINT('Ctrl Pts',(-6.13400314988651,-3.75806187938217,
-20.5247907757942));
#64580=CARTESIAN_POINT('Ctrl Pts',(-6.19164793481474,-3.71718369216096,
-20.4736489647519));
#64581=CARTESIAN_POINT('Ctrl Pts',(-6.22260859132108,-3.70420972323454,
-20.4445304195459));
#64582=CARTESIAN_POINT('Ctrl Pts',(-6.25150607875357,-3.69905785638952,
-20.4160958798464));
#64583=CARTESIAN_POINT('Ctrl Pts',(-6.2801544416415,-3.69395040366473,-20.3879064736302));
#64584=CARTESIAN_POINT('Ctrl Pts',(-6.31086688890514,-3.69580208067255,
-20.3563629124601));
#64585=CARTESIAN_POINT('Ctrl Pts',(-6.36807510645317,-3.71571514780993,
-20.2945810740561));
#64586=CARTESIAN_POINT('Ctrl Pts',(-6.39456832517073,-3.73377436649843,
-20.2643397343447));
#64587=CARTESIAN_POINT('Ctrl Pts',(-6.43496570369138,-3.77614009919508,
-20.2153893012592));
#64588=CARTESIAN_POINT('Ctrl Pts',(-6.45415498120474,-3.80533050967996,
-20.1903979662949));
#64589=CARTESIAN_POINT('Ctrl Pts',(-6.48727536023424,-3.8791679039915,-20.1426530305365));
#64590=CARTESIAN_POINT('Ctrl Pts',(-6.5,-3.94295127275524,-20.117318872842));
#64591=CARTESIAN_POINT('Ctrl Pts',(-6.5,-4.,-20.1059692628831));
#64592=CARTESIAN_POINT('Origin',(-6.,-4.,-20.1059692628831));
#64593=CARTESIAN_POINT('Origin',(11.6,-4.,-20.1059692628831));
#64594=CARTESIAN_POINT('',(11.6,-3.5,-20.1059692628831));
#64595=CARTESIAN_POINT('Origin',(-6.5,-3.5,-18.));
#64596=CARTESIAN_POINT('Origin',(-6.,0.,0.));
#64597=CARTESIAN_POINT('Origin',(-6.5,0.,0.));
#64598=CARTESIAN_POINT('Origin',(-6.35355339059327,-1.11022302462516E-15,
-1.11022302462516E-15));
#64599=CARTESIAN_POINT('Origin',(-6.5,20.5,0.));
#64600=CARTESIAN_POINT('',(-6.5,4.,-18.5741756210067));
#64601=CARTESIAN_POINT('',(-6.5,4.,-10.75));
#64602=CARTESIAN_POINT('Origin',(-6.5,0.,0.));
#64603=CARTESIAN_POINT('Origin',(-6.,4.,-10.75));
#64604=CARTESIAN_POINT('',(-6.,3.5,-18.5741756210067));
#64605=CARTESIAN_POINT('',(-6.,3.5,-10.75));
#64606=CARTESIAN_POINT('Origin',(-6.,4.,-18.5741756210067));
#64607=CARTESIAN_POINT('Origin',(-6.,4.,-18.5741756210067));
#64608=CARTESIAN_POINT('Origin',(-6.,4.,-18.5741756210067));
#64609=CARTESIAN_POINT('Origin',(-6.,4.,-18.5741756210067));
#64610=CARTESIAN_POINT('Origin',(-6.,18.5741756210067,-4.));
#64611=CARTESIAN_POINT('Origin',(-6.,18.5741756210067,-4.));
#64612=CARTESIAN_POINT('Origin',(-6.,18.5741756210067,-4.));
#64613=CARTESIAN_POINT('Origin',(5.75,18.5741756210067,-4.));
#64614=CARTESIAN_POINT('Origin',(-6.,0.,0.));
#64615=CARTESIAN_POINT('Origin',(5.75,4.,-18.5741756210067));
#64616=CARTESIAN_POINT('',(5.75,3.5,-18.5741756210067));
#64617=CARTESIAN_POINT('Origin',(-6.5,3.5,-21.5));
#64618=CARTESIAN_POINT('Origin',(-6.5,20.5,0.));
#64619=CARTESIAN_POINT('',(-6.5,-20.1975426238546,-3.50845720475184));
#64620=CARTESIAN_POINT('Origin',(-6.5,0.,0.));
#64621=CARTESIAN_POINT('',(-6.5,-20.1059692628831,-3.5));
#64622=CARTESIAN_POINT('Origin',(-6.5,-20.1059692628831,-3.99999999999999));
#64623=CARTESIAN_POINT('',(-6.5,-0.5,-3.5));
#64624=CARTESIAN_POINT('Origin',(11.6,-20.1059692628831,-3.99999999999999));
#64625=CARTESIAN_POINT('Ctrl Pts',(-6.5,-20.1975426238546,-3.50845720475183));
#64626=CARTESIAN_POINT('Ctrl Pts',(-6.44146838187229,-20.2550884935232,
-3.51917787596606));
#64627=CARTESIAN_POINT('Ctrl Pts',(-6.37838919138939,-20.3152794800863,
-3.54130503996253));
#64628=CARTESIAN_POINT('Ctrl Pts',(-6.2559198324237,-20.4273638888019,-3.6111352406743));
#64629=CARTESIAN_POINT('Ctrl Pts',(-6.19673011624031,-20.4788885029216,
-3.65972871821816));
#64630=CARTESIAN_POINT('Ctrl Pts',(-6.10742473363203,-20.5506848087795,
-3.76440047785072));
#64631=CARTESIAN_POINT('Ctrl Pts',(-6.06891141762746,-20.5788865473403,
-3.82410317982267));
#64632=CARTESIAN_POINT('Ctrl Pts',(-6.02857797268264,-20.6012039162238,
-3.92325195833915));
#64633=CARTESIAN_POINT('Ctrl Pts',(-6.01793177509303,-20.6054227657767,
-3.95789306108273));
#64634=CARTESIAN_POINT('Ctrl Pts',(-6.00364389418785,-20.6064145558324,
-4.02788015641737));
#64635=CARTESIAN_POINT('Ctrl Pts',(-6.,-20.6031896256267,-4.0632256674496));
#64636=CARTESIAN_POINT('Ctrl Pts',(-6.,-20.5963587570998,-4.09756097560975));
#64637=CARTESIAN_POINT('',(11.6,-20.1059692628831,-3.5));
#64638=CARTESIAN_POINT('Origin',(-6.5,-21.5,-3.5));
#64639=CARTESIAN_POINT('Origin',(5.75,11.145178817862,15.3878195049812));
#64640=CARTESIAN_POINT('',(7.9947148353915,11.4987322083171,15.0342661142498));
#64641=CARTESIAN_POINT('Ctrl Pts',(7.99471483544825,11.4987322084552,15.034266114388));
#64642=CARTESIAN_POINT('Ctrl Pts',(7.98790837769307,11.4656035153935,15.0011374213262));
#64643=CARTESIAN_POINT('Ctrl Pts',(7.97481356608163,11.4290648513116,14.9738935230493));
#64644=CARTESIAN_POINT('Ctrl Pts',(7.93533857113774,11.3448695865394,14.926398354714));
#64645=CARTESIAN_POINT('Ctrl Pts',(7.9072623646401,11.2974038150965,14.9091857104132));
#64646=CARTESIAN_POINT('Ctrl Pts',(7.83244151643846,11.1875808446044,14.8854247099832));
#64647=CARTESIAN_POINT('Ctrl Pts',(7.78233548373286,11.1255843049717,14.8848332489223));
#64648=CARTESIAN_POINT('Ctrl Pts',(7.65786764210673,10.9886851823176,14.9061789600546));
#64649=CARTESIAN_POINT('Ctrl Pts',(7.57955614016674,10.9156732068678,14.9371191012641));
#64650=CARTESIAN_POINT('Ctrl Pts',(7.50156833754672,10.8531390412775,14.9819705581587));
#64651=CARTESIAN_POINT('Ctrl Pts',(7.50078416818792,10.8525113125737,14.9824229952701));
#64652=CARTESIAN_POINT('Ctrl Pts',(7.5,10.8518846384445,14.9828768864291));
#64653=CARTESIAN_POINT('',(5.75,11.4987322084552,15.034266114388));
#64654=CARTESIAN_POINT('Origin',(8.,12.0208152801713,15.556349186104));
#64655=CARTESIAN_POINT('',(8.,11.5504536489008,15.0859875548336));
#64656=CARTESIAN_POINT('Ctrl Pts',(7.99471483541929,11.4987322083143,15.034266114247));
#64657=CARTESIAN_POINT('Ctrl Pts',(7.99834499874643,11.5164011002136,15.0519350061464));
#64658=CARTESIAN_POINT('Ctrl Pts',(8.,11.5339910288095,15.0695249347422));
#64659=CARTESIAN_POINT('Ctrl Pts',(8.,11.5504536489008,15.0859875548336));
#64660=CARTESIAN_POINT('',(8.,12.0208152801713,15.556349186104));
#64661=CARTESIAN_POINT('',(8.,12.0208152801713,15.556349186104));
#64662=CARTESIAN_POINT('',(29.337248848077,12.0208152801996,15.5563491860757));
#64663=CARTESIAN_POINT('',(8.,12.0208152801713,15.556349186104));
#64664=CARTESIAN_POINT('',(29.6961037355001,12.622503406322,16.1580373122142));
#64665=CARTESIAN_POINT('Ctrl Pts',(29.3372488480671,12.0208152801713,15.556349186104));
#64666=CARTESIAN_POINT('Ctrl Pts',(29.3635470277544,12.0208152801713,15.556349186104));
#64667=CARTESIAN_POINT('Ctrl Pts',(29.3897411711777,12.0223153633463,15.5578483797216));
#64668=CARTESIAN_POINT('Ctrl Pts',(29.415607431348,12.0252248665426,15.5607573876018));
#64669=CARTESIAN_POINT('Ctrl Pts',(29.4419059568771,12.0281829920537,15.5637150095193));
#64670=CARTESIAN_POINT('Ctrl Pts',(29.4678668567866,12.0325981572608,15.5681303086097));
#64671=CARTESIAN_POINT('Ctrl Pts',(29.4932488211205,12.0384121343065,15.5739465388115));
#64672=CARTESIAN_POINT('Ctrl Pts',(29.5056295238234,12.0412480504074,15.5767835539469));
#64673=CARTESIAN_POINT('Ctrl Pts',(29.5178722688888,12.0444173222899,15.5799544093235));
#64674=CARTESIAN_POINT('Ctrl Pts',(29.5299470752204,12.0479161878527,15.583455268391));
#64675=CARTESIAN_POINT('Ctrl Pts',(29.5545920296324,12.055057452062,15.5906006013887));
#64676=CARTESIAN_POINT('Ctrl Pts',(29.5783543573571,12.0635161276847,15.599065190727));
#64677=CARTESIAN_POINT('Ctrl Pts',(29.6010013147649,12.0732271832776,15.6087800031479));
#64678=CARTESIAN_POINT('Ctrl Pts',(29.6182267197699,12.0806134675631,15.6161691448982));
#64679=CARTESIAN_POINT('Ctrl Pts',(29.6348068591577,12.0887250603625,15.6242823638422));
#64680=CARTESIAN_POINT('Ctrl Pts',(29.6506294743871,12.0975465693583,15.6331010316835));
#64681=CARTESIAN_POINT('Ctrl Pts',(29.6654204617391,12.1057929196669,15.6413447260799));
#64682=CARTESIAN_POINT('Ctrl Pts',(29.6795495016601,12.11465988999,15.6502051489654));
#64683=CARTESIAN_POINT('Ctrl Pts',(29.6929623869925,12.1240948005673,15.6596335337303));
#64684=CARTESIAN_POINT('Ctrl Pts',(29.7117060225708,12.1372794749451,15.6728090887094));
#64685=CARTESIAN_POINT('Ctrl Pts',(29.7289079510306,12.1514701038323,15.6869909142991));
#64686=CARTESIAN_POINT('Ctrl Pts',(29.7444572669056,12.1664988608128,15.702017054101));
#64687=CARTESIAN_POINT('Ctrl Pts',(29.7600106951658,12.1815315925043,15.7170471679217));
#64688=CARTESIAN_POINT('Ctrl Pts',(29.7739113767554,12.1974036551567,15.7329229380823));
#64689=CARTESIAN_POINT('Ctrl Pts',(29.7860080855976,12.2139724871026,15.7495003064955));
#64690=CARTESIAN_POINT('Ctrl Pts',(29.791664963973,12.2217206993116,15.7572525106794));
#64691=CARTESIAN_POINT('Ctrl Pts',(29.7969266990531,12.2296215756952,15.7651583175465));
#64692=CARTESIAN_POINT('Ctrl Pts',(29.8017740895476,12.2376617310126,15.7732035029928));
#64693=CARTESIAN_POINT('Ctrl Pts',(29.8121759038628,12.2549147670066,15.790467332932));
#64694=CARTESIAN_POINT('Ctrl Pts',(29.8205897043332,12.2726701275567,15.8082344070815));
#64695=CARTESIAN_POINT('Ctrl Pts',(29.8268838981186,12.2907815683395,15.8263459586653));
#64696=CARTESIAN_POINT('Ctrl Pts',(29.8272913784438,12.2919540863824,15.8275184838813));
#64697=CARTESIAN_POINT('Ctrl Pts',(29.8276899587999,12.2931281037408,15.8286924566032));
#64698=CARTESIAN_POINT('Ctrl Pts',(29.8280795964848,12.2943035834062,15.8298678350682));
#64699=CARTESIAN_POINT('Ctrl Pts',(29.8341018209758,12.3124717501507,15.8480344376629));
#64700=CARTESIAN_POINT('Ctrl Pts',(29.8379920903211,12.3309885244332,15.8665369818169));
#64701=CARTESIAN_POINT('Ctrl Pts',(29.8397834073069,12.3496695928917,15.8852056233943));
#64702=CARTESIAN_POINT('Ctrl Pts',(29.8404573868658,12.3566983088467,15.8922296637593));
#64703=CARTESIAN_POINT('Ctrl Pts',(29.8408337073171,12.3637503539871,15.8992771857621));
#64704=CARTESIAN_POINT('Ctrl Pts',(29.8409122430702,12.3708160009656,15.9063388639076));
#64705=CARTESIAN_POINT('Ctrl Pts',(29.841120187594,12.3895242012339,15.9250365556235));
#64706=CARTESIAN_POINT('Ctrl Pts',(29.8392425388124,12.408176797555,15.9436833457277));
#64707=CARTESIAN_POINT('Ctrl Pts',(29.8353415852943,12.4265962129204,15.9621050094994));
#64708=CARTESIAN_POINT('Ctrl Pts',(29.8314529329103,12.444957545128,15.9804685830232));
#64709=CARTESIAN_POINT('Ctrl Pts',(29.8255535219378,12.4630881464923,15.9986093924684));
#64710=CARTESIAN_POINT('Ctrl Pts',(29.8176551502899,12.4808142028984,16.0163472264152));
#64711=CARTESIAN_POINT('Ctrl Pts',(29.8141109427822,12.4887683515505,16.0243066599602));
#64712=CARTESIAN_POINT('Ctrl Pts',(29.8101635813264,12.4966409819043,16.0321847640837));
#64713=CARTESIAN_POINT('Ctrl Pts',(29.8058109922455,12.5044157250982,16.0399639788116));
#64714=CARTESIAN_POINT('Ctrl Pts',(29.8017570288636,12.5116570528749,16.047209471336));
#64715=CARTESIAN_POINT('Ctrl Pts',(29.7973617576496,12.5187951035663,16.0543508658078));
#64716=CARTESIAN_POINT('Ctrl Pts',(29.7926271891834,12.5258177264801,16.0613748908172));
#64717=CARTESIAN_POINT('Ctrl Pts',(29.7829544505439,12.5401649677324,16.0757249965551));
#64718=CARTESIAN_POINT('Ctrl Pts',(29.7718670650361,12.5540309525854,16.0895860215957));
#64719=CARTESIAN_POINT('Ctrl Pts',(29.7594824084562,12.5673324817764,16.1028820334627));
#64720=CARTESIAN_POINT('Ctrl Pts',(29.7449214392347,12.5829714424452,16.1185145072673));
#64721=CARTESIAN_POINT('Ctrl Pts',(29.7286275829089,12.5977667684327,16.1333027723117));
#64722=CARTESIAN_POINT('Ctrl Pts',(29.7107932614126,12.6115882202006,16.1471218329623));
#64723=CARTESIAN_POINT('Ctrl Pts',(29.7060063962345,12.6152980011526,16.1508309721205));
#64724=CARTESIAN_POINT('Ctrl Pts',(29.701108313897,12.6189375257568,16.1544701493208));
#64725=CARTESIAN_POINT('Ctrl Pts',(29.6961022501539,12.622504030493,16.1580366171471));
#64726=CARTESIAN_POINT('',(29.8535533905933,12.5103262255613,16.0458601314941));
#64727=CARTESIAN_POINT('Ctrl Pts',(29.6961037355001,12.622503406322,16.1580373122142));
#64728=CARTESIAN_POINT('Ctrl Pts',(29.7751366074575,12.5661986334316,16.101732539364));
#64729=CARTESIAN_POINT('Ctrl Pts',(29.8535533905933,12.5103262255613,16.0458601314941));
#64730=CARTESIAN_POINT('',(30.,12.2583832540376,15.7939171599704));
#64731=CARTESIAN_POINT('Ctrl Pts',(29.8535533905933,12.5103262255613,16.0458601314941));
#64732=CARTESIAN_POINT('Ctrl Pts',(29.8971736290481,12.4792465554081,16.0147804613409));
#64733=CARTESIAN_POINT('Ctrl Pts',(29.9381460122713,12.4355437242224,15.9710776301552));
#64734=CARTESIAN_POINT('Ctrl Pts',(29.985486770529,12.3543653386467,15.8898992445794));
#64735=CARTESIAN_POINT('Ctrl Pts',(30.,12.3024682657458,15.8380021716785));
#64736=CARTESIAN_POINT('Ctrl Pts',(30.,12.2583832540376,15.7939171599704));
#64737=CARTESIAN_POINT('',(30.,11.5504536489008,15.0859875548336));
#64738=CARTESIAN_POINT('',(30.,9.75152416360247,13.2870580695352));
#64739=CARTESIAN_POINT('',(29.5,11.1937144438494,14.7292483497821));
#64740=CARTESIAN_POINT('Ctrl Pts',(29.5,11.1937144438494,14.7292483497821));
#64741=CARTESIAN_POINT('Ctrl Pts',(29.5615281526734,11.1937144438494,14.7292483497821));
#64742=CARTESIAN_POINT('Ctrl Pts',(29.6339241856893,11.2039672958034,14.7395012017362));
#64743=CARTESIAN_POINT('Ctrl Pts',(29.7477912665658,11.237498416831,14.7730323227637));
#64744=CARTESIAN_POINT('Ctrl Pts',(29.8093392860887,11.2667800757207,14.8023139816534));
#64745=CARTESIAN_POINT('Ctrl Pts',(29.8967622377582,11.3289413274527,14.8644752333855));
#64746=CARTESIAN_POINT('Ctrl Pts',(29.9380095827943,11.3728886696422,14.908422575575));
#64747=CARTESIAN_POINT('Ctrl Pts',(29.9854746058202,11.4543428055946,14.9898767115274));
#64748=CARTESIAN_POINT('Ctrl Pts',(30.,11.5063099570288,15.0418438629615));
#64749=CARTESIAN_POINT('Ctrl Pts',(30.,11.5504536489008,15.0859875548336));
#64750=CARTESIAN_POINT('',(25.5,11.1937144438494,14.7292483497821));
#64751=CARTESIAN_POINT('Origin',(7.5,0.,0.));
#64752=CARTESIAN_POINT('',(7.99471483561596,15.0342661152043,11.4987322092715));
#64753=CARTESIAN_POINT('',(8.,15.0859875548336,11.5504536489008));
#64754=CARTESIAN_POINT('Ctrl Pts',(8.,15.0859875548336,11.5504536489008));
#64755=CARTESIAN_POINT('Ctrl Pts',(8.,15.0695249350393,11.5339910291066));
#64756=CARTESIAN_POINT('Ctrl Pts',(7.99834499880831,15.0519350067816,11.5164011008489));
#64757=CARTESIAN_POINT('Ctrl Pts',(7.99471483561601,15.0342661152045,11.4987322092718));
#64758=CARTESIAN_POINT('Origin',(8.,0.,0.));
#64759=CARTESIAN_POINT('Ctrl Pts',(7.99471483561596,15.0342661152043,11.4987322092715));
#64760=CARTESIAN_POINT('Ctrl Pts',(7.99136258232187,15.0179498789986,11.4824159731412));
#64761=CARTESIAN_POINT('Ctrl Pts',(7.98645003622417,15.0029056934867,11.4651126007181));
#64762=CARTESIAN_POINT('Ctrl Pts',(7.96402271105946,14.9546388364367,11.4013638075551));
#64763=CARTESIAN_POINT('Ctrl Pts',(7.9393863219916,14.9298917928097,11.3524620624821));
#64764=CARTESIAN_POINT('Ctrl Pts',(7.86974221714271,14.8917374983038,11.2381679470131));
#64765=CARTESIAN_POINT('Ctrl Pts',(7.8185631647191,14.8836497863555,11.1692008513272));
#64766=CARTESIAN_POINT('Ctrl Pts',(7.68155929436919,14.8978112789661,11.011515252604));
#64767=CARTESIAN_POINT('Ctrl Pts',(7.59305526458688,14.9294271056729,10.9265492041609));
#64768=CARTESIAN_POINT('Ctrl Pts',(7.50190235999017,14.9817779053809,10.8534064745168));
#64769=CARTESIAN_POINT('Ctrl Pts',(7.5009511789491,14.9823263263295,10.8526447805273));
#64770=CARTESIAN_POINT('Ctrl Pts',(7.5,14.9828768864291,10.8518846384445));
#64771=CARTESIAN_POINT('Origin',(8.,13.3643181644258,13.3643181644258));
#64772=CARTESIAN_POINT('',(8.,15.556349186104,12.0208152801713));
#64773=CARTESIAN_POINT('',(8.,14.7078210486802,11.1722871427475));
#64774=CARTESIAN_POINT('',(8.,15.556349186104,12.0208152801713));
#64775=CARTESIAN_POINT('Origin',(28.9928932188134,0.,0.));
#64776=CARTESIAN_POINT('',(29.3464466094067,-2.55382374106385E-15,20.8535533905933));
#64777=CARTESIAN_POINT('',(29.3464466094067,-20.8535533905933,-2.55382374106385E-15));
#64778=CARTESIAN_POINT('Origin',(29.3464466094067,0.,-3.19227967632981E-15));
#64779=CARTESIAN_POINT('Origin',(29.3464466094067,0.,-3.19227967632981E-15));
#64780=CARTESIAN_POINT('Origin',(28.9928932188134,-2.51052593825207E-15,
20.5));
#64781=CARTESIAN_POINT('Origin',(29.6,0.,0.));
#64782=CARTESIAN_POINT('',(29.8535533905933,12.5103262255613,-16.0458601314941));
#64783=CARTESIAN_POINT('',(29.6961037355001,12.622503406322,-16.1580373122142));
#64784=CARTESIAN_POINT('Ctrl Pts',(29.8535533905933,12.5103262255613,-16.0458601314941));
#64785=CARTESIAN_POINT('Ctrl Pts',(29.775136607461,12.5661986334541,-16.1017325393463));
#64786=CARTESIAN_POINT('Ctrl Pts',(29.6961037355001,12.622503406322,-16.1580373122142));
#64787=CARTESIAN_POINT('',(29.8535533905933,-20.3464466094067,-2.49172107142325E-15));
#64788=CARTESIAN_POINT('Origin',(29.8535533905933,0.,-3.11465133927906E-15));
#64789=CARTESIAN_POINT('',(29.6,-20.6,-2.52277240624355E-15));
#64790=CARTESIAN_POINT('',(29.8535533905933,-16.0458601314941,12.5103262255613));
#64791=CARTESIAN_POINT('Origin',(29.8535533905933,0.,-3.11465133927906E-15));
#64792=CARTESIAN_POINT('',(29.6961037355001,-16.1580373122142,12.622503406322));
#64793=CARTESIAN_POINT('Ctrl Pts',(29.6961037355001,-16.1580373122142,12.622503406322));
#64794=CARTESIAN_POINT('Ctrl Pts',(29.7751366074575,-16.101732539364,12.5661986334316));
#64795=CARTESIAN_POINT('Ctrl Pts',(29.8535533905933,-16.0458601314941,12.5103262255613));
#64796=CARTESIAN_POINT('',(29.6961037355001,-12.622503406322,16.1580373122142));
#64797=CARTESIAN_POINT('Ctrl Pts',(29.6961021613978,-12.622503505457,16.1580371399984));
#64798=CARTESIAN_POINT('Ctrl Pts',(29.8947432207477,-13.7975614582838,14.9878688132478));
#64799=CARTESIAN_POINT('Ctrl Pts',(29.8947432207477,-14.9878688132478,13.7975614582838));
#64800=CARTESIAN_POINT('Ctrl Pts',(29.6961021613978,-16.1580371399984,12.622503505457));
#64801=CARTESIAN_POINT('',(29.8535533905933,-12.5103262255613,16.0458601314941));
#64802=CARTESIAN_POINT('Ctrl Pts',(29.8535533905933,-12.5103262255613,16.0458601314941));
#64803=CARTESIAN_POINT('Ctrl Pts',(29.775136607461,-12.5661986334541,16.1017325393463));
#64804=CARTESIAN_POINT('Ctrl Pts',(29.6961037355001,-12.622503406322,16.1580373122142));
#64805=CARTESIAN_POINT('Origin',(29.8535533905933,0.,-3.11465133927906E-15));
#64806=CARTESIAN_POINT('',(29.6961037355001,16.1580373122142,12.622503406322));
#64807=CARTESIAN_POINT('Ctrl Pts',(29.6961021613978,16.1580371399984,12.622503505457));
#64808=CARTESIAN_POINT('Ctrl Pts',(29.89474322789,14.9878687711962,13.7975615005113));
#64809=CARTESIAN_POINT('Ctrl Pts',(29.8947432136049,13.7975614160535,14.9878688553023));
#64810=CARTESIAN_POINT('Ctrl Pts',(29.6961021613977,12.622503505457,16.1580371399984));
#64811=CARTESIAN_POINT('',(29.8535533905933,16.0458601314941,12.5103262255613));
#64812=CARTESIAN_POINT('Ctrl Pts',(29.8535533905933,16.0458601314941,12.5103262255613));
#64813=CARTESIAN_POINT('Ctrl Pts',(29.775136607461,16.1017325393463,12.5661986334541));
#64814=CARTESIAN_POINT('Ctrl Pts',(29.6961037355001,16.1580373122142,12.622503406322));
#64815=CARTESIAN_POINT('',(29.8535533905933,16.0458601314941,-12.5103262255613));
#64816=CARTESIAN_POINT('Origin',(29.8535533905933,0.,-3.11465133927906E-15));
#64817=CARTESIAN_POINT('',(29.6961037355001,16.1580373122142,-12.622503406322));
#64818=CARTESIAN_POINT('Ctrl Pts',(29.6961037355001,16.1580373122142,-12.622503406322));
#64819=CARTESIAN_POINT('Ctrl Pts',(29.7751366074575,16.101732539364,-12.5661986334316));
#64820=CARTESIAN_POINT('Ctrl Pts',(29.8535533905933,16.0458601314941,-12.5103262255613));
#64821=CARTESIAN_POINT('Ctrl Pts',(29.6961021613978,12.622503505457,-16.1580371399984));
#64822=CARTESIAN_POINT('Ctrl Pts',(29.8947432207477,13.7975614582838,-14.9878688132478));
#64823=CARTESIAN_POINT('Ctrl Pts',(29.8947432207477,14.9878688132478,-13.7975614582838));
#64824=CARTESIAN_POINT('Ctrl Pts',(29.6961021613978,16.1580371399984,-12.622503505457));
#64825=CARTESIAN_POINT('Origin',(5.75,-11.145178817862,15.3878195049812));
#64826=CARTESIAN_POINT('',(5.75,-11.4987322084552,15.034266114388));
#64827=CARTESIAN_POINT('Origin',(8.,-11.1722871427475,14.7078210486802));
#64828=CARTESIAN_POINT('',(29.5,-11.1937144438494,14.7292483497821));
#64829=CARTESIAN_POINT('',(25.5,-11.1937144438494,14.7292483497821));
#64830=CARTESIAN_POINT('',(30.,-11.5504536489008,15.0859875548336));
#64831=CARTESIAN_POINT('Ctrl Pts',(30.,-11.5504536489008,15.0859875548336));
#64832=CARTESIAN_POINT('Ctrl Pts',(30.,-11.5063099570288,15.0418438629615));
#64833=CARTESIAN_POINT('Ctrl Pts',(29.9854746058202,-11.4543428055946,14.9898767115274));
#64834=CARTESIAN_POINT('Ctrl Pts',(29.9380095827943,-11.3728886696422,14.908422575575));
#64835=CARTESIAN_POINT('Ctrl Pts',(29.8967622377582,-11.3289413274527,14.8644752333855));
#64836=CARTESIAN_POINT('Ctrl Pts',(29.8093392860887,-11.2667800757207,14.8023139816534));
#64837=CARTESIAN_POINT('Ctrl Pts',(29.7477912665658,-11.237498416831,14.7730323227637));
#64838=CARTESIAN_POINT('Ctrl Pts',(29.6339241856893,-11.2039672958034,14.7395012017362));
#64839=CARTESIAN_POINT('Ctrl Pts',(29.5615281526734,-11.1937144438494,14.7292483497821));
#64840=CARTESIAN_POINT('Ctrl Pts',(29.5,-11.1937144438494,14.7292483497821));
#64841=CARTESIAN_POINT('',(30.,-12.2583832540376,15.7939171599704));
#64842=CARTESIAN_POINT('',(30.,-0.07726009489054,3.61279400082328));
#64843=CARTESIAN_POINT('Ctrl Pts',(30.,-12.2583832540376,15.7939171599704));
#64844=CARTESIAN_POINT('Ctrl Pts',(30.,-12.3024682657458,15.8380021716785));
#64845=CARTESIAN_POINT('Ctrl Pts',(29.985486770529,-12.3543653386467,15.8898992445794));
#64846=CARTESIAN_POINT('Ctrl Pts',(29.9381460122713,-12.4355437242224,15.9710776301552));
#64847=CARTESIAN_POINT('Ctrl Pts',(29.8971736290481,-12.4792465554081,16.0147804613409));
#64848=CARTESIAN_POINT('Ctrl Pts',(29.8535533905933,-12.5103262255613,16.0458601314941));
#64849=CARTESIAN_POINT('',(29.337248848077,-12.0208152801996,15.5563491860757));
#64850=CARTESIAN_POINT('Ctrl Pts',(29.6961022501482,-12.6225040304587,16.1580366171813));
#64851=CARTESIAN_POINT('Ctrl Pts',(29.7147933690558,-12.609187786889,16.1447205114285));
#64852=CARTESIAN_POINT('Ctrl Pts',(29.7319458264551,-12.5948812492744,16.1304187761189));
#64853=CARTESIAN_POINT('Ctrl Pts',(29.7473966610106,-12.5797304055295,16.1152743170362));
#64854=CARTESIAN_POINT('Ctrl Pts',(29.7626545344491,-12.5647687764009,16.1003189928335));
#64855=CARTESIAN_POINT('Ctrl Pts',(29.7762538563399,-12.5489829561878,16.084541176273));
#64856=CARTESIAN_POINT('Ctrl Pts',(29.787997904047,-12.5324961525768,16.0680539360822));
#64857=CARTESIAN_POINT('Ctrl Pts',(29.7895746977067,-12.5302825812383,16.0658403061271));
#64858=CARTESIAN_POINT('Ctrl Pts',(29.791117976733,-12.5280563584413,16.0636138598165));
#64859=CARTESIAN_POINT('Ctrl Pts',(29.79262719669,-12.5258177707357,16.0613748467601));
#64860=CARTESIAN_POINT('Ctrl Pts',(29.7964903838824,-12.5200876030991,16.0556435903428));
#64861=CARTESIAN_POINT('Ctrl Pts',(29.8001304563093,-12.5142764177544,16.0498300026419));
#64862=CARTESIAN_POINT('Ctrl Pts',(29.8035453933447,-12.5083905632827,16.0439410198973));
#64863=CARTESIAN_POINT('Ctrl Pts',(29.8135085249837,-12.4912184917917,16.0267598216216));
#64864=CARTESIAN_POINT('Ctrl Pts',(29.8214801888626,-12.4735473689987,16.0090741392566));
#64865=CARTESIAN_POINT('Ctrl Pts',(29.8274710013099,-12.455552830915,15.9910707602896));
#64866=CARTESIAN_POINT('Ctrl Pts',(29.8335196973064,-12.4373844286454,15.9728934317156));
#64867=CARTESIAN_POINT('Ctrl Pts',(29.8375493041986,-12.4188853503994,15.954391298432));
#64868=CARTESIAN_POINT('Ctrl Pts',(29.8395211658521,-12.4002313289882,15.9357419099974));
#64869=CARTESIAN_POINT('Ctrl Pts',(29.8404142905819,-12.3917822738514,15.9272949532968));
#64870=CARTESIAN_POINT('Ctrl Pts',(29.8408845785222,-12.3833014543909,15.9188176751431));
#64871=CARTESIAN_POINT('Ctrl Pts',(29.8409249324999,-12.3748057049165,15.9103263965022));
#64872=CARTESIAN_POINT('Ctrl Pts',(29.8410141353611,-12.3560257678752,15.8915563422819));
#64873=CARTESIAN_POINT('Ctrl Pts',(29.839005150545,-12.3373242933743,15.8728698715399));
#64874=CARTESIAN_POINT('Ctrl Pts',(29.8348849951903,-12.3188838478478,15.8544395081246));
#64875=CARTESIAN_POINT('Ctrl Pts',(29.8330414088442,-12.3106325683061,15.8461927398794));
#64876=CARTESIAN_POINT('Ctrl Pts',(29.8307744497582,-12.3024335569624,15.8379971208758));
#64877=CARTESIAN_POINT('Ctrl Pts',(29.828079594041,-12.2943035691538,15.8298678492748));
#64878=CARTESIAN_POINT('Ctrl Pts',(29.8221302029723,-12.2763551214691,15.8119209827503));
#64879=CARTESIAN_POINT('Ctrl Pts',(29.8140982090173,-12.2587417299286,15.7942966939978));
#64880=CARTESIAN_POINT('Ctrl Pts',(29.8041111241459,-12.2416040578225,15.777148298582));
#64881=CARTESIAN_POINT('Ctrl Pts',(29.7940809428845,-12.2243924330255,15.759925904202));
#64882=CARTESIAN_POINT('Ctrl Pts',(29.782158514763,-12.2077969859203,15.7433200368196));
#64883=CARTESIAN_POINT('Ctrl Pts',(29.7685166509587,-12.1919504656349,15.7274696634267));
#64884=CARTESIAN_POINT('Ctrl Pts',(29.7547832062128,-12.1759975640465,15.7115128828639));
#64885=CARTESIAN_POINT('Ctrl Pts',(29.7393064495632,-12.1608029018257,15.6963208650584));
#64886=CARTESIAN_POINT('Ctrl Pts',(29.7222165154168,-12.1465218786284,15.6820468667118));
#64887=CARTESIAN_POINT('Ctrl Pts',(29.714456352485,-12.1400371803322,15.6755653582456));
#64888=CARTESIAN_POINT('Ctrl Pts',(29.7063630119465,-12.133741204959,15.6692733727736));
#64889=CARTESIAN_POINT('Ctrl Pts',(29.6979461657047,-12.1276505214833,15.663186817225));
#64890=CARTESIAN_POINT('Ctrl Pts',(29.6830664509242,-12.1168831116564,15.6524267049506));
#64891=CARTESIAN_POINT('Ctrl Pts',(29.6672686286642,-12.106823322986,15.6423747899711));
#64892=CARTESIAN_POINT('Ctrl Pts',(29.6506294745141,-12.0975465700894,15.6331010309531));
#64893=CARTESIAN_POINT('Ctrl Pts',(29.6298333664988,-12.0859522093709,15.6215104120729));
#64894=CARTESIAN_POINT('Ctrl Pts',(29.6077235557432,-12.0755796101762,15.6111339862795));
#64895=CARTESIAN_POINT('Ctrl Pts',(29.5845492431071,-12.0664699003604,15.6020196611318));
#64896=CARTESIAN_POINT('Ctrl Pts',(29.5693077818247,-12.0604785559079,15.5960252812322));
#64897=CARTESIAN_POINT('Ctrl Pts',(29.5536050740522,-12.0550341298654,15.5905773505175));
#64898=CARTESIAN_POINT('Ctrl Pts',(29.5375065797936,-12.0501564727128,15.5856968465475));
#64899=CARTESIAN_POINT('Ctrl Pts',(29.5129698031991,-12.042722113826,15.5782581486383));
#64900=CARTESIAN_POINT('Ctrl Pts',(29.4876554246782,-12.0366454880391,15.5721786672796));
#64901=CARTESIAN_POINT('Ctrl Pts',(29.4618081716839,-12.0319809750165,15.5675131353444));
#64902=CARTESIAN_POINT('Ctrl Pts',(29.4544053482885,-12.030645027783,15.5661768962876));
#64903=CARTESIAN_POINT('Ctrl Pts',(29.4469586955947,-12.0294251369375,15.564956850236));
#64904=CARTESIAN_POINT('Ctrl Pts',(29.4394737482924,-12.0283231275853,15.5638548093301));
#64905=CARTESIAN_POINT('Ctrl Pts',(29.4134898262845,-12.0244975128009,15.5600290850074));
#64906=CARTESIAN_POINT('Ctrl Pts',(29.3871445400212,-12.0221044238458,15.5576374033428));
#64907=CARTESIAN_POINT('Ctrl Pts',(29.3606723115461,-12.0212111743809,15.5567447799941));
#64908=CARTESIAN_POINT('Ctrl Pts',(29.3528735776467,-12.0209480225692,15.5564818126367));
#64909=CARTESIAN_POINT('Ctrl Pts',(29.3450637756841,-12.0208152801713,15.556349186104));
#64910=CARTESIAN_POINT('Ctrl Pts',(29.3372488480671,-12.0208152801713,15.556349186104));
#64911=CARTESIAN_POINT('',(8.,-12.0208152801713,15.556349186104));
#64912=CARTESIAN_POINT('Origin',(5.75,15.3878195049812,11.145178817862));
#64913=CARTESIAN_POINT('',(5.75,15.034266114388,11.4987322084552));
#64914=CARTESIAN_POINT('Origin',(8.,14.7078210486802,11.1722871427475));
#64915=CARTESIAN_POINT('',(29.5,14.7292483497821,11.1937144438494));
#64916=CARTESIAN_POINT('',(25.5,14.7292483497821,11.1937144438494));
#64917=CARTESIAN_POINT('',(30.,15.0859875548336,11.5504536489008));
#64918=CARTESIAN_POINT('Ctrl Pts',(30.,15.0859875548336,11.5504536489008));
#64919=CARTESIAN_POINT('Ctrl Pts',(30.,15.0418438629615,11.5063099570288));
#64920=CARTESIAN_POINT('Ctrl Pts',(29.9854746058202,14.9898767115274,11.4543428055946));
#64921=CARTESIAN_POINT('Ctrl Pts',(29.9380095827943,14.908422575575,11.3728886696422));
#64922=CARTESIAN_POINT('Ctrl Pts',(29.8967622377582,14.8644752333855,11.3289413274527));
#64923=CARTESIAN_POINT('Ctrl Pts',(29.8093392860887,14.8023139816534,11.2667800757207));
#64924=CARTESIAN_POINT('Ctrl Pts',(29.7477912665658,14.7730323227637,11.237498416831));
#64925=CARTESIAN_POINT('Ctrl Pts',(29.6339241856893,14.7395012017362,11.2039672958034));
#64926=CARTESIAN_POINT('Ctrl Pts',(29.5615281526734,14.7292483497821,11.1937144438494));
#64927=CARTESIAN_POINT('Ctrl Pts',(29.5,14.7292483497821,11.1937144438494));
#64928=CARTESIAN_POINT('',(30.,15.7939171599704,12.2583832540376));
#64929=CARTESIAN_POINT('',(30.,12.8627940008233,9.32726009489054));
#64930=CARTESIAN_POINT('Ctrl Pts',(30.,15.7939171599704,12.2583832540376));
#64931=CARTESIAN_POINT('Ctrl Pts',(30.,15.8380021716785,12.3024682657458));
#64932=CARTESIAN_POINT('Ctrl Pts',(29.985486770529,15.8898992445794,12.3543653386467));
#64933=CARTESIAN_POINT('Ctrl Pts',(29.9381460122713,15.9710776301552,12.4355437242224));
#64934=CARTESIAN_POINT('Ctrl Pts',(29.8971736290481,16.0147804613409,12.4792465554081));
#64935=CARTESIAN_POINT('Ctrl Pts',(29.8535533905933,16.0458601314941,12.5103262255613));
#64936=CARTESIAN_POINT('',(29.337248848077,15.5563491860757,12.0208152801996));
#64937=CARTESIAN_POINT('Ctrl Pts',(29.6961022501425,16.1580366172154,12.6225040304245));
#64938=CARTESIAN_POINT('Ctrl Pts',(29.7147933690495,16.1447205114661,12.6091877868512));
#64939=CARTESIAN_POINT('Ctrl Pts',(29.7319458264482,16.1304187761599,12.5948812492331));
#64940=CARTESIAN_POINT('Ctrl Pts',(29.7473966610032,16.1152743170805,12.5797304054849));
#64941=CARTESIAN_POINT('Ctrl Pts',(29.7626545344412,16.1003189928811,12.5647687763529));
#64942=CARTESIAN_POINT('Ctrl Pts',(29.7762538563314,16.0845411763236,12.5489829561367));
#64943=CARTESIAN_POINT('Ctrl Pts',(29.787997904038,16.0680539361356,12.532496152523));
#64944=CARTESIAN_POINT('Ctrl Pts',(29.7895746976977,16.0658403061808,12.5302825811841));
#64945=CARTESIAN_POINT('Ctrl Pts',(29.7911179767239,16.0636138598707,12.5280563583868));
#64946=CARTESIAN_POINT('Ctrl Pts',(29.7926271966808,16.0613748468147,12.5258177706809));
#64947=CARTESIAN_POINT('Ctrl Pts',(29.7964903838731,16.0556435903983,12.5200876030434));
#64948=CARTESIAN_POINT('Ctrl Pts',(29.8001304562998,16.0498300026983,12.5142764176978));
#64949=CARTESIAN_POINT('Ctrl Pts',(29.8035453933351,16.0439410199545,12.5083905632253));
#64950=CARTESIAN_POINT('Ctrl Pts',(29.8135085249737,16.0267598216811,12.4912184917317));
#64951=CARTESIAN_POINT('Ctrl Pts',(29.8214801888522,16.0090741393181,12.4735473689368));
#64952=CARTESIAN_POINT('Ctrl Pts',(29.8274710012993,15.9910707603526,12.4555528308514));
#64953=CARTESIAN_POINT('Ctrl Pts',(29.8335196972955,15.97289343178,12.4373844285801));
#64954=CARTESIAN_POINT('Ctrl Pts',(29.8375493041875,15.9543912984974,12.418885350333));
#64955=CARTESIAN_POINT('Ctrl Pts',(29.8395211658409,15.9357419100632,12.4002313289212));
#64956=CARTESIAN_POINT('Ctrl Pts',(29.8404142905707,15.9272949533631,12.3917822737844));
#64957=CARTESIAN_POINT('Ctrl Pts',(29.8408845785109,15.9188176752096,12.3833014543239));
#64958=CARTESIAN_POINT('Ctrl Pts',(29.8409249324886,15.9103263965689,12.3748057048496));
#64959=CARTESIAN_POINT('Ctrl Pts',(29.8410141353498,15.8915563423485,12.3560257678082));
#64960=CARTESIAN_POINT('Ctrl Pts',(29.8390051505338,15.8728698716057,12.3373242933078));
#64961=CARTESIAN_POINT('Ctrl Pts',(29.8348849951791,15.8544395081892,12.3188838477822));
#64962=CARTESIAN_POINT('Ctrl Pts',(29.8330414088332,15.8461927399437,12.3106325682411));
#64963=CARTESIAN_POINT('Ctrl Pts',(29.8307744497472,15.8379971209396,12.3024335568982));
#64964=CARTESIAN_POINT('Ctrl Pts',(29.8280795940302,15.829867849338,12.2943035690904));
#64965=CARTESIAN_POINT('Ctrl Pts',(29.8221302029618,15.8119209828121,12.2763551214071));
#64966=CARTESIAN_POINT('Ctrl Pts',(29.8140982090071,15.7942966940576,12.2587417298686));
#64967=CARTESIAN_POINT('Ctrl Pts',(29.8041111241361,15.7771482986394,12.2416040577649));
#64968=CARTESIAN_POINT('Ctrl Pts',(29.7940809428751,15.759925904257,12.2243924329705));
#64969=CARTESIAN_POINT('Ctrl Pts',(29.7821585147542,15.7433200368719,12.2077969858681));
#64970=CARTESIAN_POINT('Ctrl Pts',(29.7685166509504,15.727469663476,12.1919504655859));
#64971=CARTESIAN_POINT('Ctrl Pts',(29.7547832062051,15.7115128829102,12.1759975640006));
#64972=CARTESIAN_POINT('Ctrl Pts',(29.7393064495563,15.6963208651015,12.1608029017832));
#64973=CARTESIAN_POINT('Ctrl Pts',(29.7222165154105,15.6820468667515,12.1465218785895));
#64974=CARTESIAN_POINT('Ctrl Pts',(29.7144563524789,15.6755653582836,12.1400371802947));
#64975=CARTESIAN_POINT('Ctrl Pts',(29.7063630119405,15.6692733728098,12.1337412049229));
#64976=CARTESIAN_POINT('Ctrl Pts',(29.6979461656987,15.6631868172595,12.1276505214487));
#64977=CARTESIAN_POINT('Ctrl Pts',(29.6830664509188,15.6524267049823,12.1168831116246));
#64978=CARTESIAN_POINT('Ctrl Pts',(29.6672686286593,15.6423747899999,12.1068233229571));
#64979=CARTESIAN_POINT('Ctrl Pts',(29.6506294745096,15.6331010309793,12.0975465700633));
#64980=CARTESIAN_POINT('Ctrl Pts',(29.629833366495,15.6215104120956,12.0859522093482));
#64981=CARTESIAN_POINT('Ctrl Pts',(29.60772355574,15.6111339862989,12.0755796101569));
#64982=CARTESIAN_POINT('Ctrl Pts',(29.5845492431045,15.6020196611483,12.0664699003441));
#64983=CARTESIAN_POINT('Ctrl Pts',(29.5693077818223,15.5960252812466,12.0604785558936));
#64984=CARTESIAN_POINT('Ctrl Pts',(29.5536050740501,15.59057735053,12.0550341298529));
#64985=CARTESIAN_POINT('Ctrl Pts',(29.5375065797918,15.5856968465582,12.0501564727021));
#64986=CARTESIAN_POINT('Ctrl Pts',(29.5129698031983,15.5782581486466,12.042722113818));
#64987=CARTESIAN_POINT('Ctrl Pts',(29.4876554246784,15.5721786672858,12.0366454880335));
#64988=CARTESIAN_POINT('Ctrl Pts',(29.4618081716851,15.567513135349,12.0319809750126));
#64989=CARTESIAN_POINT('Ctrl Pts',(29.4544053482892,15.5661768962915,12.0306450277795));
#64990=CARTESIAN_POINT('Ctrl Pts',(29.4469586955948,15.5649568502393,12.0294251369344));
#64991=CARTESIAN_POINT('Ctrl Pts',(29.4394737482919,15.5638548093329,12.0283231275825));
#64992=CARTESIAN_POINT('Ctrl Pts',(29.4134898262827,15.5600290850086,12.0244975127992));
#64993=CARTESIAN_POINT('Ctrl Pts',(29.387144540018,15.557637403343,12.022104423845));
#64994=CARTESIAN_POINT('Ctrl Pts',(29.3606723115413,15.5567447799941,12.0212111743806));
#64995=CARTESIAN_POINT('Ctrl Pts',(29.3528735776436,15.5564818126367,12.0209480225691));
#64996=CARTESIAN_POINT('Ctrl Pts',(29.3450637756825,15.556349186104,12.0208152801713));
#64997=CARTESIAN_POINT('Ctrl Pts',(29.3372488480671,15.556349186104,12.0208152801713));
#64998=CARTESIAN_POINT('',(8.,15.556349186104,12.0208152801713));
#64999=CARTESIAN_POINT('Origin',(5.75,11.145178817862,-15.3878195049812));
#65000=CARTESIAN_POINT('',(5.75,11.4987322084552,-15.034266114388));
#65001=CARTESIAN_POINT('Origin',(8.,11.1722871427474,-14.7078210486802));
#65002=CARTESIAN_POINT('',(29.5,11.1937144438493,-14.7292483497821));
#65003=CARTESIAN_POINT('',(25.5,11.1937144438493,-14.7292483497821));
#65004=CARTESIAN_POINT('',(30.,11.5504536489008,-15.0859875548336));
#65005=CARTESIAN_POINT('Ctrl Pts',(30.,11.5504536489008,-15.0859875548336));
#65006=CARTESIAN_POINT('Ctrl Pts',(30.,11.5063099570288,-15.0418438629615));
#65007=CARTESIAN_POINT('Ctrl Pts',(29.9854746058202,11.4543428055946,-14.9898767115274));
#65008=CARTESIAN_POINT('Ctrl Pts',(29.9380095827943,11.3728886696422,-14.908422575575));
#65009=CARTESIAN_POINT('Ctrl Pts',(29.8967622377582,11.3289413274527,-14.8644752333855));
#65010=CARTESIAN_POINT('Ctrl Pts',(29.8093392860887,11.2667800757207,-14.8023139816534));
#65011=CARTESIAN_POINT('Ctrl Pts',(29.7477912665658,11.237498416831,-14.7730323227637));
#65012=CARTESIAN_POINT('Ctrl Pts',(29.6339241856893,11.2039672958034,-14.7395012017362));
#65013=CARTESIAN_POINT('Ctrl Pts',(29.5615281526734,11.1937144438494,-14.7292483497821));
#65014=CARTESIAN_POINT('Ctrl Pts',(29.5,11.1937144438494,-14.7292483497821));
#65015=CARTESIAN_POINT('',(30.,12.2583832540376,-15.7939171599704));
#65016=CARTESIAN_POINT('',(30.,9.32726009489054,-12.8627940008233));
#65017=CARTESIAN_POINT('Ctrl Pts',(30.,12.2583832540376,-15.7939171599704));
#65018=CARTESIAN_POINT('Ctrl Pts',(30.,12.3024682657458,-15.8380021716785));
#65019=CARTESIAN_POINT('Ctrl Pts',(29.985486770529,12.3543653386467,-15.8898992445794));
#65020=CARTESIAN_POINT('Ctrl Pts',(29.9381460122713,12.4355437242224,-15.9710776301552));
#65021=CARTESIAN_POINT('Ctrl Pts',(29.8971736290481,12.4792465554081,-16.0147804613409));
#65022=CARTESIAN_POINT('Ctrl Pts',(29.8535533905933,12.5103262255613,-16.0458601314941));
#65023=CARTESIAN_POINT('',(29.337248848077,12.0208152801996,-15.5563491860757));
#65024=CARTESIAN_POINT('Ctrl Pts',(29.6961022501482,12.6225040304587,-16.1580366171813));
#65025=CARTESIAN_POINT('Ctrl Pts',(29.7147933690559,12.6091877868889,-16.1447205114284));
#65026=CARTESIAN_POINT('Ctrl Pts',(29.7319458264552,12.5948812492743,-16.1304187761187));
#65027=CARTESIAN_POINT('Ctrl Pts',(29.7473966610108,12.5797304055293,-16.115274317036));
#65028=CARTESIAN_POINT('Ctrl Pts',(29.7626545344494,12.5647687764006,-16.1003189928333));
#65029=CARTESIAN_POINT('Ctrl Pts',(29.7762538563401,12.5489829561875,-16.0845411762727));
#65030=CARTESIAN_POINT('Ctrl Pts',(29.7879979040472,12.5324961525765,-16.0680539360819));
#65031=CARTESIAN_POINT('Ctrl Pts',(29.7895746977069,12.530282581238,-16.0658403061268));
#65032=CARTESIAN_POINT('Ctrl Pts',(29.7911179767331,12.5280563584412,-16.0636138598164));
#65033=CARTESIAN_POINT('Ctrl Pts',(29.79262719669,12.5258177707357,-16.0613748467601));
#65034=CARTESIAN_POINT('Ctrl Pts',(29.7964903838824,12.5200876030991,-16.0556435903428));
#65035=CARTESIAN_POINT('Ctrl Pts',(29.8001304563093,12.5142764177544,-16.0498300026419));
#65036=CARTESIAN_POINT('Ctrl Pts',(29.8035453933447,12.5083905632827,-16.0439410198973));
#65037=CARTESIAN_POINT('Ctrl Pts',(29.8135085249837,12.4912184917917,-16.0267598216216));
#65038=CARTESIAN_POINT('Ctrl Pts',(29.8214801888625,12.4735473689988,-16.0090741392567));
#65039=CARTESIAN_POINT('Ctrl Pts',(29.8274710013099,12.4555528309151,-15.9910707602897));
#65040=CARTESIAN_POINT('Ctrl Pts',(29.8335196973064,12.4373844286455,-15.9728934317157));
#65041=CARTESIAN_POINT('Ctrl Pts',(29.8375493041985,12.4188853503995,-15.9543912984321));
#65042=CARTESIAN_POINT('Ctrl Pts',(29.8395211658521,12.4002313289884,-15.9357419099975));
#65043=CARTESIAN_POINT('Ctrl Pts',(29.8404142905819,12.3917822738516,-15.927294953297));
#65044=CARTESIAN_POINT('Ctrl Pts',(29.8408845785222,12.3833014543909,-15.9188176751432));
#65045=CARTESIAN_POINT('Ctrl Pts',(29.8409249324999,12.3748057049165,-15.9103263965022));
#65046=CARTESIAN_POINT('Ctrl Pts',(29.8410141353611,12.356025767875,-15.8915563422818));
#65047=CARTESIAN_POINT('Ctrl Pts',(29.839005150545,12.3373242933741,-15.8728698715396));
#65048=CARTESIAN_POINT('Ctrl Pts',(29.8348849951902,12.3188838478474,-15.8544395081242));
#65049=CARTESIAN_POINT('Ctrl Pts',(29.8330414088442,12.3106325683058,-15.8461927398792));
#65050=CARTESIAN_POINT('Ctrl Pts',(29.8307744497581,12.3024335569623,-15.8379971208756));
#65051=CARTESIAN_POINT('Ctrl Pts',(29.828079594041,12.2943035691539,-15.8298678492748));
#65052=CARTESIAN_POINT('Ctrl Pts',(29.8221302029723,12.2763551214691,-15.8119209827503));
#65053=CARTESIAN_POINT('Ctrl Pts',(29.8140982090173,12.2587417299286,-15.7942966939978));
#65054=CARTESIAN_POINT('Ctrl Pts',(29.8041111241459,12.2416040578225,-15.777148298582));
#65055=CARTESIAN_POINT('Ctrl Pts',(29.7940809428845,12.2243924330256,-15.759925904202));
#65056=CARTESIAN_POINT('Ctrl Pts',(29.7821585147631,12.2077969859204,-15.7433200368197));
#65057=CARTESIAN_POINT('Ctrl Pts',(29.7685166509588,12.1919504656351,-15.7274696634269));
#65058=CARTESIAN_POINT('Ctrl Pts',(29.754783206213,12.1759975640467,-15.7115128828641));
#65059=CARTESIAN_POINT('Ctrl Pts',(29.7393064495636,12.160802901826,-15.6963208650588));
#65060=CARTESIAN_POINT('Ctrl Pts',(29.7222165154172,12.1465218786288,-15.6820468667122));
#65061=CARTESIAN_POINT('Ctrl Pts',(29.7144563524853,12.1400371803324,-15.6755653582458));
#65062=CARTESIAN_POINT('Ctrl Pts',(29.7063630119467,12.1337412049591,-15.6692733727737));
#65063=CARTESIAN_POINT('Ctrl Pts',(29.6979461657046,12.1276505214833,-15.663186817225));
#65064=CARTESIAN_POINT('Ctrl Pts',(29.6830664509242,12.1168831116564,-15.6524267049506));
#65065=CARTESIAN_POINT('Ctrl Pts',(29.6672686286642,12.106823322986,-15.6423747899711));
#65066=CARTESIAN_POINT('Ctrl Pts',(29.6506294745141,12.0975465700894,-15.6331010309531));
#65067=CARTESIAN_POINT('Ctrl Pts',(29.6298333664989,12.085952209371,-15.6215104120729));
#65068=CARTESIAN_POINT('Ctrl Pts',(29.6077235557434,12.0755796101763,-15.6111339862796));
#65069=CARTESIAN_POINT('Ctrl Pts',(29.5845492431074,12.0664699003605,-15.602019661132));
#65070=CARTESIAN_POINT('Ctrl Pts',(29.5693077818249,12.060478555908,-15.5960252812323));
#65071=CARTESIAN_POINT('Ctrl Pts',(29.5536050740523,12.0550341298654,-15.5905773505176));
#65072=CARTESIAN_POINT('Ctrl Pts',(29.5375065797936,12.0501564727128,-15.5856968465475));
#65073=CARTESIAN_POINT('Ctrl Pts',(29.5129698031991,12.042722113826,-15.5782581486383));
#65074=CARTESIAN_POINT('Ctrl Pts',(29.4876554246782,12.0366454880391,-15.5721786672796));
#65075=CARTESIAN_POINT('Ctrl Pts',(29.4618081716839,12.0319809750165,-15.5675131353444));
#65076=CARTESIAN_POINT('Ctrl Pts',(29.4544053482885,12.0306450277829,-15.5661768962876));
#65077=CARTESIAN_POINT('Ctrl Pts',(29.4469586955947,12.0294251369375,-15.564956850236));
#65078=CARTESIAN_POINT('Ctrl Pts',(29.4394737482924,12.0283231275853,-15.5638548093301));
#65079=CARTESIAN_POINT('Ctrl Pts',(29.413489826283,12.0244975128006,-15.5600290850072));
#65080=CARTESIAN_POINT('Ctrl Pts',(29.3871445400181,12.0221044238455,-15.5576374033425));
#65081=CARTESIAN_POINT('Ctrl Pts',(29.3606723115414,12.0212111743808,-15.556744779994));
#65082=CARTESIAN_POINT('Ctrl Pts',(29.3528735776436,12.0209480225692,-15.5564818126366));
#65083=CARTESIAN_POINT('Ctrl Pts',(29.3450637756825,12.0208152801713,-15.556349186104));
#65084=CARTESIAN_POINT('Ctrl Pts',(29.3372488480671,12.0208152801713,-15.556349186104));
#65085=CARTESIAN_POINT('',(8.,12.0208152801713,-15.556349186104));
#65086=CARTESIAN_POINT('Origin',(29.5,-0.147970773009215,-4.39061146012847));
#65087=CARTESIAN_POINT('',(29.988172366943,-12.0208153231845,-16.1105655469847));
#65088=CARTESIAN_POINT('',(30.,-11.8557283302283,-16.0983690173476));
#65089=CARTESIAN_POINT('Ctrl Pts',(29.9881723667624,-12.0208153202678,-16.1105655869574));
#65090=CARTESIAN_POINT('Ctrl Pts',(29.9959139993979,-11.9675244706852,-16.1067121202485));
#65091=CARTESIAN_POINT('Ctrl Pts',(29.9997996576908,-11.913571858627,-16.1027290501183));
#65092=CARTESIAN_POINT('Ctrl Pts',(29.9999974820111,-11.8585310768755,-16.0985804389105));
#65093=CARTESIAN_POINT('Ctrl Pts',(30.,-11.8571296997207,-16.0984747560115));
#65094=CARTESIAN_POINT('Ctrl Pts',(30.,-11.8557283302283,-16.0983690173476));
#65095=CARTESIAN_POINT('',(30.,-11.145178817862,-15.3878195049812));
#65096=CARTESIAN_POINT('',(30.,-0.147970773009215,-4.39061146012847));
#65097=CARTESIAN_POINT('',(29.5,-11.4987322084552,-15.034266114388));
#65098=CARTESIAN_POINT('Origin',(29.5,-11.145178817862,-15.3878195049812));
#65099=CARTESIAN_POINT('',(29.5,-12.0208152801713,-15.556349186104));
#65100=CARTESIAN_POINT('',(29.5,-0.501524163602491,-4.0370580695352));
#65101=CARTESIAN_POINT('Origin',(29.5,-12.0208152801713,-16.2634559672906));
#65102=CARTESIAN_POINT('Origin',(29.5,0.,0.));
#65103=CARTESIAN_POINT('',(29.5,-10.8518846384445,-14.9828768864291));
#65104=CARTESIAN_POINT('Origin',(29.5,0.,0.));
#65105=CARTESIAN_POINT('Origin',(29.5,-11.145178817862,-15.3878195049812));
#65106=CARTESIAN_POINT('Origin',(30.,0.,0.));
#65107=CARTESIAN_POINT('Origin',(29.5,-11.145178817862,-15.3878195049812));
#65108=CARTESIAN_POINT('Origin',(29.5,-11.145178817862,-15.3878195049812));
#65109=CARTESIAN_POINT('Origin',(25.5,-11.145178817862,-15.3878195049812));
#65110=CARTESIAN_POINT('',(25.5,-10.8518846384445,-14.9828768864291));
#65111=CARTESIAN_POINT('',(25.5,-11.4987322084552,-15.034266114388));
#65112=CARTESIAN_POINT('Origin',(25.5,0.,0.));
#65113=CARTESIAN_POINT('Origin',(30.,18.5,0.));
#65114=CARTESIAN_POINT('Origin',(30.,0.,0.));
#65115=CARTESIAN_POINT('Ctrl Pts',(29.3372488480671,15.556349186104,-12.0208152801713));
#65116=CARTESIAN_POINT('Ctrl Pts',(29.5429564710669,14.3836353036043,-13.1935291626711));
#65117=CARTESIAN_POINT('Ctrl Pts',(29.5429564710669,13.1935291626711,-14.3836353036043));
#65118=CARTESIAN_POINT('Ctrl Pts',(29.3372488480671,12.0208152801713,-15.556349186104));
#65119=CARTESIAN_POINT('Ctrl Pts',(29.4482318142554,15.5660830361542,-12.0110814301211));
#65120=CARTESIAN_POINT('Ctrl Pts',(29.6555084018099,14.3871511086965,-13.1900026135806));
#65121=CARTESIAN_POINT('Ctrl Pts',(29.6555084018099,13.1900026135806,-14.3871511086965));
#65122=CARTESIAN_POINT('Ctrl Pts',(29.4482318142554,12.0110814301211,-15.5660830361542));
#65123=CARTESIAN_POINT('Ctrl Pts',(29.6698854043403,15.640712881006,-12.0468306632344));
#65124=CARTESIAN_POINT('Ctrl Pts',(29.8803030333723,14.449846680584,-13.2386772974356));
#65125=CARTESIAN_POINT('Ctrl Pts',(29.8803030333723,13.2386772974356,-14.449846680584));
#65126=CARTESIAN_POINT('Ctrl Pts',(29.6698854043403,12.0468306632344,-15.640712881006));
#65127=CARTESIAN_POINT('Ctrl Pts',(29.8584164372574,15.8692592876068,-12.2423065389736));
#65128=CARTESIAN_POINT('Ctrl Pts',(30.070315495024,14.6693103047466,-13.446404317352));
#65129=CARTESIAN_POINT('Ctrl Pts',(30.070315495024,13.446404317352,-14.6693103047466));
#65130=CARTESIAN_POINT('Ctrl Pts',(29.8584164372574,12.2423065389736,-15.8692592876068));
#65131=CARTESIAN_POINT('Ctrl Pts',(29.826995289044,16.074348363723,-12.4529072490931));
#65132=CARTESIAN_POINT('Ctrl Pts',(30.0363416090412,14.876799813501,-13.6562728118144));
#65133=CARTESIAN_POINT('Ctrl Pts',(30.0363416090412,13.6562728118144,-14.876799813501));
#65134=CARTESIAN_POINT('Ctrl Pts',(29.826995289044,12.4529072490931,-16.074348363723));
#65135=CARTESIAN_POINT('Ctrl Pts',(29.7297376388611,16.1642229909118,-12.5598419966883));
#65136=CARTESIAN_POINT('Ctrl Pts',(29.9363897461384,14.9718056381716,-13.7576323115672));
#65137=CARTESIAN_POINT('Ctrl Pts',(29.9363897461384,13.7576323115672,-14.9718056381716));
#65138=CARTESIAN_POINT('Ctrl Pts',(29.7297376388611,12.5598419966883,-16.1642229909118));
#65139=CARTESIAN_POINT('Ctrl Pts',(29.6908022386604,16.188980729523,-12.5914294562957));
#65140=CARTESIAN_POINT('Ctrl Pts',(29.8965098616602,14.9985443441187,-13.7869294139585));
#65141=CARTESIAN_POINT('Ctrl Pts',(29.8965098616602,13.7869294139585,-14.9985443441187));
#65142=CARTESIAN_POINT('Ctrl Pts',(29.6908022386603,12.5914294562957,-16.188980729523));
#65143=CARTESIAN_POINT('',(29.337248848077,15.5563491860757,-12.0208152801996));
#65144=CARTESIAN_POINT('Ctrl Pts',(29.3372488480671,15.556349186104,-12.0208152801713));
#65145=CARTESIAN_POINT('Ctrl Pts',(29.3635470277545,15.556349186104,-12.0208152801713));
#65146=CARTESIAN_POINT('Ctrl Pts',(29.3897411711777,15.5578483797221,-12.0223153633457));
#65147=CARTESIAN_POINT('Ctrl Pts',(29.4156074313478,15.5607573876035,-12.025224866541));
#65148=CARTESIAN_POINT('Ctrl Pts',(29.4419059568767,15.5637150095221,-12.028182992051));
#65149=CARTESIAN_POINT('Ctrl Pts',(29.467866856786,15.5681303086141,-12.0325981572563));
#65150=CARTESIAN_POINT('Ctrl Pts',(29.4932488211195,15.5739465388181,-12.0384121343));
#65151=CARTESIAN_POINT('Ctrl Pts',(29.5056295238222,15.5767835539545,-12.0412480503998));
#65152=CARTESIAN_POINT('Ctrl Pts',(29.5178722688873,15.5799544093323,-12.0444173222812));
#65153=CARTESIAN_POINT('Ctrl Pts',(29.5299470752187,15.583455268401,-12.0479161878428));
#65154=CARTESIAN_POINT('Ctrl Pts',(29.5545920296303,15.5906006014012,-12.0550574520495));
#65155=CARTESIAN_POINT('Ctrl Pts',(29.5783543573545,15.5990651907424,-12.0635161276693));
#65156=CARTESIAN_POINT('Ctrl Pts',(29.6010013147618,15.6087800031665,-12.0732271832591));
#65157=CARTESIAN_POINT('Ctrl Pts',(29.6182267197664,15.6161691449192,-12.0806134675421));
#65158=CARTESIAN_POINT('Ctrl Pts',(29.6348068591537,15.6242823638657,-12.088725060339));
#65159=CARTESIAN_POINT('Ctrl Pts',(29.6506294743827,15.6331010317096,-12.0975465693321));
#65160=CARTESIAN_POINT('Ctrl Pts',(29.6654204617342,15.6413447261084,-12.1057929196383));
#65161=CARTESIAN_POINT('Ctrl Pts',(29.6795495016548,15.6502051489965,-12.1146598899589));
#65162=CARTESIAN_POINT('Ctrl Pts',(29.6929623869868,15.6596335337639,-12.1240948005337));
#65163=CARTESIAN_POINT('Ctrl Pts',(29.7117060225645,15.6728090887466,-12.137279474908));
#65164=CARTESIAN_POINT('Ctrl Pts',(29.7289079510238,15.6869909143398,-12.1514701037918));
#65165=CARTESIAN_POINT('Ctrl Pts',(29.7444572668983,15.702017054145,-12.166498860769));
#65166=CARTESIAN_POINT('Ctrl Pts',(29.7600106951579,15.7170471679691,-12.1815315924573));
#65167=CARTESIAN_POINT('Ctrl Pts',(29.7739113767471,15.7329229381329,-12.1974036551066));
#65168=CARTESIAN_POINT('Ctrl Pts',(29.7860080855888,15.749500306549,-12.2139724870497));
#65169=CARTESIAN_POINT('Ctrl Pts',(29.7916649639638,15.757252510734,-12.2217206992573));
#65170=CARTESIAN_POINT('Ctrl Pts',(29.7969266990437,15.7651583176022,-12.2296215756395));
#65171=CARTESIAN_POINT('Ctrl Pts',(29.8017740895379,15.7732035030496,-12.2376617309556));
#65172=CARTESIAN_POINT('Ctrl Pts',(29.8121759038527,15.7904673329913,-12.2549147669471));
#65173=CARTESIAN_POINT('Ctrl Pts',(29.8205897043228,15.8082344071429,-12.2726701274951));
#65174=CARTESIAN_POINT('Ctrl Pts',(29.8268838981079,15.8263459587283,-12.2907815682763));
#65175=CARTESIAN_POINT('Ctrl Pts',(29.827291378433,15.8275184839444,-12.2919540863191));
#65176=CARTESIAN_POINT('Ctrl Pts',(29.8276899587891,15.8286924566664,-12.2931281036774));
#65177=CARTESIAN_POINT('Ctrl Pts',(29.828079596474,15.8298678351315,-12.2943035833427));
#65178=CARTESIAN_POINT('Ctrl Pts',(29.8341018209648,15.8480344377277,-12.3124717500857));
#65179=CARTESIAN_POINT('Ctrl Pts',(29.8379920903099,15.8665369818828,-12.3309885243672));
#65180=CARTESIAN_POINT('Ctrl Pts',(29.8397834072957,15.8852056234607,-12.3496695928252));
#65181=CARTESIAN_POINT('Ctrl Pts',(29.8404573868545,15.8922296638259,-12.35669830878));
#65182=CARTESIAN_POINT('Ctrl Pts',(29.8408337073058,15.8992771858287,-12.3637503539203));
#65183=CARTESIAN_POINT('Ctrl Pts',(29.8409122430589,15.9063388639742,-12.3708160008987));
#65184=CARTESIAN_POINT('Ctrl Pts',(29.8411201875827,15.9250365556903,-12.3895242011671));
#65185=CARTESIAN_POINT('Ctrl Pts',(29.8392425388012,15.9436833457942,-12.4081767974889));
#65186=CARTESIAN_POINT('Ctrl Pts',(29.8353415852832,15.9621050095651,-12.4265962128555));
#65187=CARTESIAN_POINT('Ctrl Pts',(29.8314529328993,15.9804685830881,-12.4449575450642));
#65188=CARTESIAN_POINT('Ctrl Pts',(29.8255535219269,15.9986093925319,-12.4630881464303));
#65189=CARTESIAN_POINT('Ctrl Pts',(29.8176551502792,16.0163472264769,-12.4808142028385));
#65190=CARTESIAN_POINT('Ctrl Pts',(29.8141109427718,16.0243066600206,-12.4887683514911));
#65191=CARTESIAN_POINT('Ctrl Pts',(29.8101635813163,16.0321847641428,-12.4966409818456));
#65192=CARTESIAN_POINT('Ctrl Pts',(29.8058109922358,16.0399639788694,-12.5044157250402));
#65193=CARTESIAN_POINT('Ctrl Pts',(29.801757028854,16.0472094713927,-12.5116570528179));
#65194=CARTESIAN_POINT('Ctrl Pts',(29.7973617576402,16.0543508658634,-12.5187951035103));
#65195=CARTESIAN_POINT('Ctrl Pts',(29.7926271891742,16.0613748908717,-12.5258177264253));
#65196=CARTESIAN_POINT('Ctrl Pts',(29.7829544505351,16.0757249966074,-12.5401649676799));
#65197=CARTESIAN_POINT('Ctrl Pts',(29.7718670650277,16.0895860216454,-12.5540309525354));
#65198=CARTESIAN_POINT('Ctrl Pts',(29.7594824084483,16.1028820335097,-12.5673324817292));
#65199=CARTESIAN_POINT('Ctrl Pts',(29.7449214392272,16.1185145073112,-12.5829714424013));
#65200=CARTESIAN_POINT('Ctrl Pts',(29.7286275829019,16.1333027723524,-12.5977667683923));
#65201=CARTESIAN_POINT('Ctrl Pts',(29.7107932614059,16.1471218329996,-12.6115882201639));
#65202=CARTESIAN_POINT('Ctrl Pts',(29.7060063962282,16.1508309721568,-12.6152980011167));
#65203=CARTESIAN_POINT('Ctrl Pts',(29.7011083138909,16.1544701493559,-12.6189375257217));
#65204=CARTESIAN_POINT('Ctrl Pts',(29.6961022501482,16.1580366171813,-12.6225040304587));
#65205=CARTESIAN_POINT('Ctrl Pts',(29.3372488480671,15.556349186104,-12.0208152801713));
#65206=CARTESIAN_POINT('Ctrl Pts',(29.5429564710669,14.3836353036043,-13.1935291626711));
#65207=CARTESIAN_POINT('Ctrl Pts',(29.5429564710669,13.1935291626711,-14.3836353036043));
#65208=CARTESIAN_POINT('Ctrl Pts',(29.3372488480671,12.0208152801713,-15.556349186104));
#65209=CARTESIAN_POINT('Origin',(8.,12.0208152801713,-15.556349186104));
#65210=CARTESIAN_POINT('',(8.,15.556349186104,-12.0208152801713));
#65211=CARTESIAN_POINT('Origin',(29.5,0.,0.));
#65212=CARTESIAN_POINT('',(30.,15.7939171599704,-12.2583832540376));
#65213=CARTESIAN_POINT('Ctrl Pts',(29.8535533905933,16.0458601314941,-12.5103262255613));
#65214=CARTESIAN_POINT('Ctrl Pts',(29.8971736290481,16.0147804613409,-12.4792465554081));
#65215=CARTESIAN_POINT('Ctrl Pts',(29.9381460122713,15.9710776301552,-12.4355437242224));
#65216=CARTESIAN_POINT('Ctrl Pts',(29.985486770529,15.8898992445794,-12.3543653386467));
#65217=CARTESIAN_POINT('Ctrl Pts',(30.,15.8380021716785,-12.3024682657458));
#65218=CARTESIAN_POINT('Ctrl Pts',(30.,15.7939171599704,-12.2583832540376));
#65219=CARTESIAN_POINT('Origin',(30.,0.,0.));
#65220=CARTESIAN_POINT('Origin',(30.,18.5,0.));
#65221=CARTESIAN_POINT('',(30.,15.0859875548336,-11.5504536489008));
#65222=CARTESIAN_POINT('',(30.,13.2870580695352,-9.75152416360247));
#65223=CARTESIAN_POINT('Origin',(30.,0.,0.));
#65224=CARTESIAN_POINT('Origin',(29.5,0.,0.));
#65225=CARTESIAN_POINT('',(29.5,14.7292483497821,-11.1937144438494));
#65226=CARTESIAN_POINT('Origin',(29.5,0.,0.));
#65227=CARTESIAN_POINT('Ctrl Pts',(29.5,14.7292483497821,-11.1937144438494));
#65228=CARTESIAN_POINT('Ctrl Pts',(29.5615281526734,14.7292483497821,-11.1937144438494));
#65229=CARTESIAN_POINT('Ctrl Pts',(29.6339241856893,14.7395012017362,-11.2039672958035));
#65230=CARTESIAN_POINT('Ctrl Pts',(29.7477912665658,14.7730323227637,-11.237498416831));
#65231=CARTESIAN_POINT('Ctrl Pts',(29.8093392860887,14.8023139816534,-11.2667800757207));
#65232=CARTESIAN_POINT('Ctrl Pts',(29.8967622377582,14.8644752333855,-11.3289413274527));
#65233=CARTESIAN_POINT('Ctrl Pts',(29.9380095827943,14.908422575575,-11.3728886696422));
#65234=CARTESIAN_POINT('Ctrl Pts',(29.9854746058202,14.9898767115274,-11.4543428055946));
#65235=CARTESIAN_POINT('Ctrl Pts',(30.,15.0418438629615,-11.5063099570288));
#65236=CARTESIAN_POINT('Ctrl Pts',(30.,15.0859875548336,-11.5504536489008));
#65237=CARTESIAN_POINT('Ctrl Pts',(29.3372488480671,12.0208152801713,15.556349186104));
#65238=CARTESIAN_POINT('Ctrl Pts',(29.5429564635396,13.1935291197589,14.3836353465164));
#65239=CARTESIAN_POINT('Ctrl Pts',(29.5429564785937,14.383635260695,13.1935292055803));
#65240=CARTESIAN_POINT('Ctrl Pts',(29.3372488480671,15.556349186104,12.0208152801713));
#65241=CARTESIAN_POINT('Ctrl Pts',(29.4482318142554,12.0110814301211,15.5660830361542));
#65242=CARTESIAN_POINT('Ctrl Pts',(29.6555083942252,13.1900025704413,14.3871511518362));
#65243=CARTESIAN_POINT('Ctrl Pts',(29.6555084093941,14.3871510655598,13.190002656717));
#65244=CARTESIAN_POINT('Ctrl Pts',(29.4482318142554,15.5660830361542,12.0110814301211));
#65245=CARTESIAN_POINT('Ctrl Pts',(29.6698854043403,12.0468306632344,15.640712881006));
#65246=CARTESIAN_POINT('Ctrl Pts',(29.8803030256726,13.2386772538233,14.4498467241604));
#65247=CARTESIAN_POINT('Ctrl Pts',(29.8803030410714,14.4498466370106,13.2386773410449));
#65248=CARTESIAN_POINT('Ctrl Pts',(29.6698854043403,15.640712881006,12.0468306632344));
#65249=CARTESIAN_POINT('Ctrl Pts',(29.8584164372574,12.2423065389736,15.8692592876068));
#65250=CARTESIAN_POINT('Ctrl Pts',(30.0703154872701,13.4464042732914,14.6693103486554));
#65251=CARTESIAN_POINT('Ctrl Pts',(30.0703155027773,14.6693102608408,13.4464043614096));
#65252=CARTESIAN_POINT('Ctrl Pts',(29.8584164372574,15.8692592876068,12.2423065389736));
#65253=CARTESIAN_POINT('Ctrl Pts',(29.826995289044,12.4529072490931,16.074348363723));
#65254=CARTESIAN_POINT('Ctrl Pts',(30.0363416013808,13.6562727677806,14.8767998573219));
#65255=CARTESIAN_POINT('Ctrl Pts',(30.0363416167011,14.8767997696831,13.6562728558452));
#65256=CARTESIAN_POINT('Ctrl Pts',(29.826995289044,16.074348363723,12.4529072490931));
#65257=CARTESIAN_POINT('Ctrl Pts',(29.7297376388611,12.5598419966883,16.1642229909118));
#65258=CARTESIAN_POINT('Ctrl Pts',(29.9363897385765,13.7576322677374,14.9718056818048));
#65259=CARTESIAN_POINT('Ctrl Pts',(29.9363897536997,14.9718055945414,13.7576323553939));
#65260=CARTESIAN_POINT('Ctrl Pts',(29.7297376388611,16.1642229909118,12.5598419966883));
#65261=CARTESIAN_POINT('Ctrl Pts',(29.6908022386603,12.5914294562957,16.188980729523));
#65262=CARTESIAN_POINT('Ctrl Pts',(29.8965098541329,13.7869293702126,14.9985443876794));
#65263=CARTESIAN_POINT('Ctrl Pts',(29.8965098691869,14.998544300561,13.7869294577015));
#65264=CARTESIAN_POINT('Ctrl Pts',(29.6908022386603,16.188980729523,12.5914294562957));
#65265=CARTESIAN_POINT('Ctrl Pts',(29.3372488480671,12.0208152801713,15.556349186104));
#65266=CARTESIAN_POINT('Ctrl Pts',(29.5429564635396,13.1935291197589,14.3836353465164));
#65267=CARTESIAN_POINT('Ctrl Pts',(29.5429564785937,14.383635260695,13.1935292055803));
#65268=CARTESIAN_POINT('Ctrl Pts',(29.3372488480671,15.556349186104,12.0208152801713));
#65269=CARTESIAN_POINT('Origin',(8.,15.556349186104,12.0208152801713));
#65270=CARTESIAN_POINT('Origin',(29.5,0.,0.));
#65271=CARTESIAN_POINT('Origin',(30.,0.,0.));
#65272=CARTESIAN_POINT('Origin',(30.,18.5,0.));
#65273=CARTESIAN_POINT('Origin',(30.,0.,0.));
#65274=CARTESIAN_POINT('Origin',(29.5,0.,0.));
#65275=CARTESIAN_POINT('Origin',(29.5,0.,0.));
#65276=CARTESIAN_POINT('Ctrl Pts',(29.3372488480671,-15.556349186104,12.0208152801713));
#65277=CARTESIAN_POINT('Ctrl Pts',(29.5429564710669,-14.3836353036043,13.1935291626711));
#65278=CARTESIAN_POINT('Ctrl Pts',(29.5429564710669,-13.1935291626711,14.3836353036043));
#65279=CARTESIAN_POINT('Ctrl Pts',(29.3372488480671,-12.0208152801713,15.556349186104));
#65280=CARTESIAN_POINT('Ctrl Pts',(29.4482318142553,-15.5660830361542,12.0110814301211));
#65281=CARTESIAN_POINT('Ctrl Pts',(29.6555084018099,-14.3871511086965,13.1900026135806));
#65282=CARTESIAN_POINT('Ctrl Pts',(29.6555084018099,-13.1900026135806,14.3871511086965));
#65283=CARTESIAN_POINT('Ctrl Pts',(29.4482318142553,-12.0110814301211,15.5660830361542));
#65284=CARTESIAN_POINT('Ctrl Pts',(29.6698854043403,-15.640712881006,12.0468306632344));
#65285=CARTESIAN_POINT('Ctrl Pts',(29.8803030333723,-14.449846680584,13.2386772974356));
#65286=CARTESIAN_POINT('Ctrl Pts',(29.8803030333723,-13.2386772974356,14.449846680584));
#65287=CARTESIAN_POINT('Ctrl Pts',(29.6698854043403,-12.0468306632344,15.640712881006));
#65288=CARTESIAN_POINT('Ctrl Pts',(29.8584164372574,-15.8692592876068,12.2423065389736));
#65289=CARTESIAN_POINT('Ctrl Pts',(30.070315495024,-14.6693103047466,13.446404317352));
#65290=CARTESIAN_POINT('Ctrl Pts',(30.070315495024,-13.446404317352,14.6693103047466));
#65291=CARTESIAN_POINT('Ctrl Pts',(29.8584164372574,-12.2423065389736,15.8692592876068));
#65292=CARTESIAN_POINT('Ctrl Pts',(29.826995289044,-16.074348363723,12.4529072490931));
#65293=CARTESIAN_POINT('Ctrl Pts',(30.0363416090412,-14.876799813501,13.6562728118144));
#65294=CARTESIAN_POINT('Ctrl Pts',(30.0363416090412,-13.6562728118144,14.876799813501));
#65295=CARTESIAN_POINT('Ctrl Pts',(29.826995289044,-12.4529072490931,16.074348363723));
#65296=CARTESIAN_POINT('Ctrl Pts',(29.7297376388611,-16.1642229909118,12.5598419966883));
#65297=CARTESIAN_POINT('Ctrl Pts',(29.9363897461384,-14.9718056381716,13.7576323115672));
#65298=CARTESIAN_POINT('Ctrl Pts',(29.9363897461384,-13.7576323115672,14.9718056381716));
#65299=CARTESIAN_POINT('Ctrl Pts',(29.7297376388611,-12.5598419966883,16.1642229909118));
#65300=CARTESIAN_POINT('Ctrl Pts',(29.6908022386603,-16.188980729523,12.5914294562957));
#65301=CARTESIAN_POINT('Ctrl Pts',(29.8965098616602,-14.9985443441187,13.7869294139585));
#65302=CARTESIAN_POINT('Ctrl Pts',(29.8965098616602,-13.7869294139585,14.9985443441187));
#65303=CARTESIAN_POINT('Ctrl Pts',(29.6908022386603,-12.5914294562957,16.188980729523));
#65304=CARTESIAN_POINT('',(29.337248848077,-15.5563491860757,12.0208152801996));
#65305=CARTESIAN_POINT('Ctrl Pts',(29.3372488480671,-15.556349186104,12.0208152801713));
#65306=CARTESIAN_POINT('Ctrl Pts',(29.3635470277544,-15.556349186104,12.0208152801713));
#65307=CARTESIAN_POINT('Ctrl Pts',(29.3897411711776,-15.5578483797221,12.0223153633457));
#65308=CARTESIAN_POINT('Ctrl Pts',(29.4156074313478,-15.5607573876035,12.025224866541));
#65309=CARTESIAN_POINT('Ctrl Pts',(29.4419059568766,-15.5637150095221,12.028182992051));
#65310=CARTESIAN_POINT('Ctrl Pts',(29.4678668567859,-15.5681303086141,12.0325981572563));
#65311=CARTESIAN_POINT('Ctrl Pts',(29.4932488211195,-15.5739465388181,12.0384121343));
#65312=CARTESIAN_POINT('Ctrl Pts',(29.5056295238221,-15.5767835539545,12.0412480503998));
#65313=CARTESIAN_POINT('Ctrl Pts',(29.5178722688873,-15.5799544093323,12.0444173222812));
#65314=CARTESIAN_POINT('Ctrl Pts',(29.5299470752186,-15.583455268401,12.0479161878428));
#65315=CARTESIAN_POINT('Ctrl Pts',(29.5545920296302,-15.5906006014011,12.0550574520495));
#65316=CARTESIAN_POINT('Ctrl Pts',(29.5783543573544,-15.5990651907424,12.0635161276693));
#65317=CARTESIAN_POINT('Ctrl Pts',(29.6010013147616,-15.6087800031665,12.073227183259));
#65318=CARTESIAN_POINT('Ctrl Pts',(29.6182267197663,-15.6161691449192,12.0806134675421));
#65319=CARTESIAN_POINT('Ctrl Pts',(29.6348068591536,-15.6242823638657,12.088725060339));
#65320=CARTESIAN_POINT('Ctrl Pts',(29.6506294743827,-15.6331010317096,12.0975465693321));
#65321=CARTESIAN_POINT('Ctrl Pts',(29.6654204617342,-15.6413447261084,12.1057929196383));
#65322=CARTESIAN_POINT('Ctrl Pts',(29.6795495016547,-15.6502051489965,12.1146598899589));
#65323=CARTESIAN_POINT('Ctrl Pts',(29.6929623869867,-15.6596335337639,12.1240948005337));
#65324=CARTESIAN_POINT('Ctrl Pts',(29.7117060225645,-15.6728090887465,12.137279474908));
#65325=CARTESIAN_POINT('Ctrl Pts',(29.7289079510236,-15.6869909143397,12.1514701037917));
#65326=CARTESIAN_POINT('Ctrl Pts',(29.7444572668981,-15.7020170541449,12.1664988607689));
#65327=CARTESIAN_POINT('Ctrl Pts',(29.7600106951577,-15.7170471679689,12.181531592457));
#65328=CARTESIAN_POINT('Ctrl Pts',(29.7739113767468,-15.7329229381326,12.1974036551064));
#65329=CARTESIAN_POINT('Ctrl Pts',(29.7860080855885,-15.7495003065487,12.2139724870494));
#65330=CARTESIAN_POINT('Ctrl Pts',(29.7916649639637,-15.7572525107338,12.221720699257));
#65331=CARTESIAN_POINT('Ctrl Pts',(29.7969266990436,-15.7651583176021,12.2296215756394));
#65332=CARTESIAN_POINT('Ctrl Pts',(29.8017740895379,-15.7732035030496,12.2376617309556));
#65333=CARTESIAN_POINT('Ctrl Pts',(29.8121759038527,-15.7904673329912,12.2549147669471));
#65334=CARTESIAN_POINT('Ctrl Pts',(29.8205897043228,-15.8082344071429,12.272670127495));
#65335=CARTESIAN_POINT('Ctrl Pts',(29.8268838981079,-15.8263459587282,12.2907815682763));
#65336=CARTESIAN_POINT('Ctrl Pts',(29.827291378433,-15.8275184839444,12.291954086319));
#65337=CARTESIAN_POINT('Ctrl Pts',(29.8276899587891,-15.8286924566664,12.2931281036774));
#65338=CARTESIAN_POINT('Ctrl Pts',(29.828079596474,-15.8298678351315,12.2943035833427));
#65339=CARTESIAN_POINT('Ctrl Pts',(29.8341018209648,-15.8480344377277,12.3124717500857));
#65340=CARTESIAN_POINT('Ctrl Pts',(29.8379920903099,-15.8665369818827,12.3309885243672));
#65341=CARTESIAN_POINT('Ctrl Pts',(29.8397834072957,-15.8852056234606,12.3496695928251));
#65342=CARTESIAN_POINT('Ctrl Pts',(29.8404573868545,-15.8922296638258,12.35669830878));
#65343=CARTESIAN_POINT('Ctrl Pts',(29.8408337073058,-15.8992771858287,12.3637503539203));
#65344=CARTESIAN_POINT('Ctrl Pts',(29.8409122430589,-15.9063388639742,12.3708160008987));
#65345=CARTESIAN_POINT('Ctrl Pts',(29.8411201875827,-15.9250365556902,12.389524201167));
#65346=CARTESIAN_POINT('Ctrl Pts',(29.8392425388012,-15.9436833457941,12.4081767974887));
#65347=CARTESIAN_POINT('Ctrl Pts',(29.8353415852832,-15.9621050095649,12.4265962128552));
#65348=CARTESIAN_POINT('Ctrl Pts',(29.8314529328994,-15.9804685830877,12.4449575450639));
#65349=CARTESIAN_POINT('Ctrl Pts',(29.8255535219271,-15.9986093925314,12.4630881464298));
#65350=CARTESIAN_POINT('Ctrl Pts',(29.8176551502795,-16.0163472264763,12.4808142028379));
#65351=CARTESIAN_POINT('Ctrl Pts',(29.814110942772,-16.0243066600203,12.4887683514908));
#65352=CARTESIAN_POINT('Ctrl Pts',(29.8101635813164,-16.0321847641427,12.4966409818454));
#65353=CARTESIAN_POINT('Ctrl Pts',(29.8058109922358,-16.0399639788694,12.5044157250402));
#65354=CARTESIAN_POINT('Ctrl Pts',(29.801757028854,-16.0472094713927,12.5116570528179));
#65355=CARTESIAN_POINT('Ctrl Pts',(29.7973617576402,-16.0543508658634,12.5187951035103));
#65356=CARTESIAN_POINT('Ctrl Pts',(29.7926271891742,-16.0613748908717,12.5258177264253));
#65357=CARTESIAN_POINT('Ctrl Pts',(29.7829544505351,-16.0757249966074,12.5401649676799));
#65358=CARTESIAN_POINT('Ctrl Pts',(29.7718670650277,-16.0895860216454,12.5540309525354));
#65359=CARTESIAN_POINT('Ctrl Pts',(29.7594824084483,-16.1028820335097,12.5673324817292));
#65360=CARTESIAN_POINT('Ctrl Pts',(29.7449214392259,-16.1185145073126,12.5829714424027));
#65361=CARTESIAN_POINT('Ctrl Pts',(29.728627582899,-16.133302772355,12.597766768395));
#65362=CARTESIAN_POINT('Ctrl Pts',(29.7107932614012,-16.1471218330033,12.6115882201676));
#65363=CARTESIAN_POINT('Ctrl Pts',(29.7060063962249,-16.1508309721592,12.6152980011191));
#65364=CARTESIAN_POINT('Ctrl Pts',(29.7011083138893,-16.1544701493571,12.6189375257229));
#65365=CARTESIAN_POINT('Ctrl Pts',(29.6961022501482,-16.1580366171813,12.6225040304587));
#65366=CARTESIAN_POINT('Ctrl Pts',(29.3372488480671,-15.556349186104,12.0208152801713));
#65367=CARTESIAN_POINT('Ctrl Pts',(29.5429564710669,-14.3836353036043,13.1935291626711));
#65368=CARTESIAN_POINT('Ctrl Pts',(29.5429564710669,-13.1935291626711,14.3836353036043));
#65369=CARTESIAN_POINT('Ctrl Pts',(29.3372488480671,-12.0208152801713,15.556349186104));
#65370=CARTESIAN_POINT('Origin',(8.,-12.0208152801713,15.556349186104));
#65371=CARTESIAN_POINT('',(8.,-15.556349186104,12.0208152801713));
#65372=CARTESIAN_POINT('Origin',(30.,18.5,0.));
#65373=CARTESIAN_POINT('',(30.,-15.0859875548336,11.5504536489008));
#65374=CARTESIAN_POINT('',(30.,-15.7939171599704,12.2583832540376));
#65375=CARTESIAN_POINT('',(30.,-4.03705806953519,0.501524163602477));
#65376=CARTESIAN_POINT('',(30.,-16.0983690173476,-11.8557283302283));
#65377=CARTESIAN_POINT('Origin',(30.,0.,0.));
#65378=CARTESIAN_POINT('',(30.,-15.3878195049812,-11.145178817862));
#65379=CARTESIAN_POINT('',(30.,-3.96634739141655,0.276293295702733));
#65380=CARTESIAN_POINT('Origin',(30.,0.,0.));
#65381=CARTESIAN_POINT('Origin',(29.5,0.,0.));
#65382=CARTESIAN_POINT('',(29.5,-14.7292483497821,11.1937144438494));
#65383=CARTESIAN_POINT('Ctrl Pts',(29.5,-14.7292483497821,11.1937144438494));
#65384=CARTESIAN_POINT('Ctrl Pts',(29.5615281526734,-14.7292483497821,11.1937144438494));
#65385=CARTESIAN_POINT('Ctrl Pts',(29.6339241856893,-14.7395012017362,11.2039672958034));
#65386=CARTESIAN_POINT('Ctrl Pts',(29.7477912665658,-14.7730323227637,11.237498416831));
#65387=CARTESIAN_POINT('Ctrl Pts',(29.8093392860887,-14.8023139816534,11.2667800757207));
#65388=CARTESIAN_POINT('Ctrl Pts',(29.8967622377582,-14.8644752333855,11.3289413274527));
#65389=CARTESIAN_POINT('Ctrl Pts',(29.9380095827943,-14.908422575575,11.3728886696422));
#65390=CARTESIAN_POINT('Ctrl Pts',(29.9854746058202,-14.9898767115274,11.4543428055946));
#65391=CARTESIAN_POINT('Ctrl Pts',(30.,-15.0418438629615,11.5063099570288));
#65392=CARTESIAN_POINT('Ctrl Pts',(30.,-15.0859875548336,11.5504536489008));
#65393=CARTESIAN_POINT('',(29.5,-14.9828768864291,-10.8518846384445));
#65394=CARTESIAN_POINT('Origin',(29.5,-15.3878195049812,-11.145178817862));
#65395=CARTESIAN_POINT('Origin',(29.5,0.,0.));
#65396=CARTESIAN_POINT('Origin',(29.5,-3.96634739141655,0.276293295702733));
#65397=CARTESIAN_POINT('',(29.9881723725086,-16.1105655835414,-12.0208152807707));
#65398=CARTESIAN_POINT('Ctrl Pts',(30.,-16.0983690173476,-11.8557283302283));
#65399=CARTESIAN_POINT('Ctrl Pts',(30.,-16.0984747560115,-11.8571296997209));
#65400=CARTESIAN_POINT('Ctrl Pts',(29.9999974820111,-16.0985804389106,-11.8585310768763));
#65401=CARTESIAN_POINT('Ctrl Pts',(29.9997996577384,-16.1027290491185,-11.9135718453621));
#65402=CARTESIAN_POINT('Ctrl Pts',(29.9959140013199,-16.1067121182789,-11.9675244439996));
#65403=CARTESIAN_POINT('Ctrl Pts',(29.9881723725061,-16.1105655840984,-12.02081528073));
#65404=CARTESIAN_POINT('',(29.5,-15.556349186104,-12.0208152801713));
#65405=CARTESIAN_POINT('Origin',(29.5,-16.2634559672906,-12.0208152801713));
#65406=CARTESIAN_POINT('',(29.5,-15.034266114388,-11.4987322084552));
#65407=CARTESIAN_POINT('',(29.5,-3.61279400082328,-0.0772600948905394));
#65408=CARTESIAN_POINT('Origin',(29.5,-15.3878195049812,-11.145178817862));
#65409=CARTESIAN_POINT('Origin',(29.5,-15.3878195049812,-11.145178817862));
#65410=CARTESIAN_POINT('Origin',(29.5,-15.3878195049812,-11.145178817862));
#65411=CARTESIAN_POINT('Origin',(25.5,0.,0.));
#65412=CARTESIAN_POINT('',(25.5,-14.9828768864291,-10.8518846384445));
#65413=CARTESIAN_POINT('',(25.5,-14.7292483497821,11.1937144438494));
#65414=CARTESIAN_POINT('Origin',(25.5,-15.3878195049812,-11.145178817862));
#65415=CARTESIAN_POINT('',(25.5,-15.034266114388,-11.4987322084552));
#65416=CARTESIAN_POINT('Origin',(8.,-14.7078210486802,-11.1722871427475));
#65417=CARTESIAN_POINT('',(8.,-15.556349186104,-12.0208152801713));
#65418=CARTESIAN_POINT('',(8.,-15.556349186104,-12.0208152801713));
#65419=CARTESIAN_POINT('',(8.,-15.0859875548336,-11.5504536489008));
#65420=CARTESIAN_POINT('',(8.,-14.7078210486802,-11.1722871427475));
#65421=CARTESIAN_POINT('',(7.99471483544825,-15.034266114388,-11.4987322084552));
#65422=CARTESIAN_POINT('Ctrl Pts',(7.9947148354483,-15.0342661143882,-11.4987322084555));
#65423=CARTESIAN_POINT('Ctrl Pts',(7.99834499875555,-15.05193500624,-11.5164011003073));
#65424=CARTESIAN_POINT('Ctrl Pts',(8.,-15.0695249347861,-11.5339910288533));
#65425=CARTESIAN_POINT('Ctrl Pts',(8.,-15.0859875548336,-11.5504536489008));
#65426=CARTESIAN_POINT('',(5.75,-15.034266114388,-11.4987322084552));
#65427=CARTESIAN_POINT('',(18.5,-14.7078210486802,-11.1722871427475));
#65428=CARTESIAN_POINT('Origin',(18.5,-14.3542676580869,-10.8187337521542));
#65429=CARTESIAN_POINT('',(20.5,-14.7078210486802,-11.1722871427475));
#65430=CARTESIAN_POINT('',(8.,-14.7078210486802,-11.1722871427475));
#65431=CARTESIAN_POINT('Origin',(20.5,-14.3542676580869,-10.8187337521542));
#65432=CARTESIAN_POINT('Origin',(29.5,0.,0.));
#65433=CARTESIAN_POINT('',(29.9932812305893,-12.316603510208,-15.8521374161407));
#65434=CARTESIAN_POINT('Ctrl Pts',(29.9932812305893,-12.316603510208,-15.8521374161407));
#65435=CARTESIAN_POINT('Ctrl Pts',(29.9919012225592,-12.2164522272255,-15.9405042246621));
#65436=CARTESIAN_POINT('Ctrl Pts',(29.9902210922164,-12.1178209250676,-16.0266428857885));
#65437=CARTESIAN_POINT('Ctrl Pts',(29.9881723734926,-12.0208153230367,-16.1105655469738));
#65438=CARTESIAN_POINT('',(29.9932812305893,-15.8521374161407,-12.3166035102079));
#65439=CARTESIAN_POINT('Ctrl Pts',(29.9932812305893,-12.316603510208,-15.8521374161407));
#65440=CARTESIAN_POINT('Ctrl Pts',(30.0014921231503,-12.912492379305,-15.3263648446124));
#65441=CARTESIAN_POINT('Ctrl Pts',(29.9999747373918,-13.5018717719603,-14.7749150943608));
#65442=CARTESIAN_POINT('Ctrl Pts',(29.9999996618613,-14.7028008951429,-13.5788340778648));
#65443=CARTESIAN_POINT('Ctrl Pts',(30.0020243268535,-15.2922859539755,-12.9511159833143));
#65444=CARTESIAN_POINT('Ctrl Pts',(29.9932812305893,-15.8521374161407,-12.3166035102079));
#65445=CARTESIAN_POINT('Ctrl Pts',(29.9881723725999,-16.1105655835412,-12.0208152807686));
#65446=CARTESIAN_POINT('Ctrl Pts',(29.9902249428434,-16.0264851557198,-12.1180032443948));
#65447=CARTESIAN_POINT('Ctrl Pts',(29.9919036240457,-15.940350448964,-12.2166265102365));
#65448=CARTESIAN_POINT('Ctrl Pts',(29.9932812305893,-15.8521374161407,-12.3166035102079));
#65449=CARTESIAN_POINT('Ctrl Pts',(29.8535533905933,-16.0458601314941,12.5103262255613));
#65450=CARTESIAN_POINT('Ctrl Pts',(29.8971736290481,-16.0147804613409,12.4792465554081));
#65451=CARTESIAN_POINT('Ctrl Pts',(29.9381460122713,-15.9710776301552,12.4355437242224));
#65452=CARTESIAN_POINT('Ctrl Pts',(29.985486770529,-15.8898992445794,12.3543653386467));
#65453=CARTESIAN_POINT('Ctrl Pts',(30.,-15.8380021716785,12.3024682657458));
#65454=CARTESIAN_POINT('Ctrl Pts',(30.,-15.7939171599704,12.2583832540376));
#65455=CARTESIAN_POINT('Origin',(29.5,-10.4010191002141,-17.8832521472478));
#65456=CARTESIAN_POINT('',(29.5,-10.0474657096209,-17.5296987566545));
#65457=CARTESIAN_POINT('Origin',(8.,-12.0208152801713,-15.556349186104));
#65458=CARTESIAN_POINT('',(20.5,-11.1722871427475,-14.7078210486802));
#65459=CARTESIAN_POINT('Origin',(20.5,-10.8187337521542,-14.3542676580869));
#65460=CARTESIAN_POINT('',(18.5,-11.1722871427475,-14.7078210486802));
#65461=CARTESIAN_POINT('',(8.,-11.1722871427475,-14.7078210486802));
#65462=CARTESIAN_POINT('Origin',(18.5,-10.8187337521542,-14.3542676580869));
#65463=CARTESIAN_POINT('',(7.99471483544825,-11.4987322084552,-15.034266114388));
#65464=CARTESIAN_POINT('',(5.75,-11.4987322084552,-15.034266114388));
#65465=CARTESIAN_POINT('',(8.,-11.5504536489008,-15.0859875548336));
#65466=CARTESIAN_POINT('Ctrl Pts',(8.,-11.5504536489008,-15.0859875548336));
#65467=CARTESIAN_POINT('Ctrl Pts',(8.,-11.5339910288533,-15.0695249347861));
#65468=CARTESIAN_POINT('Ctrl Pts',(7.99834499875555,-11.5164011003073,-15.05193500624));
#65469=CARTESIAN_POINT('Ctrl Pts',(7.9947148354483,-11.4987322084555,-15.0342661143882));
#65470=CARTESIAN_POINT('',(8.,-12.0208152801713,-15.556349186104));
#65471=CARTESIAN_POINT('',(8.,-12.0208152801713,-15.556349186104));
#65472=CARTESIAN_POINT('',(8.,-12.0208152801713,-15.556349186104));
#65473=CARTESIAN_POINT('Origin',(8.,-15.556349186104,-12.0208152801713));
#65474=CARTESIAN_POINT('',(8.,-15.556349186104,-12.0208152801713));
#65475=CARTESIAN_POINT('Origin',(18.5,-7.07761722863737,-18.0953841816037));
#65476=CARTESIAN_POINT('',(18.5,-7.43117061923064,-18.448937572197));
#65477=CARTESIAN_POINT('Origin',(8.,-11.1722871427475,-14.7078210486802));
#65478=CARTESIAN_POINT('',(20.5,-9.80617061923064,-16.073937572197));
#65479=CARTESIAN_POINT('Origin',(20.5,-9.45261722863737,-15.7203841816037));
#65480=CARTESIAN_POINT('Origin',(5.75,-15.3878195049812,-11.145178817862));
#65481=CARTESIAN_POINT('Ctrl Pts',(7.99471483544825,-15.034266114388,-11.4987322084552));
#65482=CARTESIAN_POINT('Ctrl Pts',(7.98769634133013,-15.0001053885364,-11.4645714826037));
#65483=CARTESIAN_POINT('Ctrl Pts',(7.97399551550773,-14.9722150037425,-11.4267999995771));
#65484=CARTESIAN_POINT('Ctrl Pts',(7.93177050929415,-14.9230460849828,-11.3379640139829));
#65485=CARTESIAN_POINT('Ctrl Pts',(7.90093775901624,-14.9057072463616,-11.2870133597151));
#65486=CARTESIAN_POINT('Ctrl Pts',(7.8176582095554,-14.8833482376701,-11.1678537278356));
#65487=CARTESIAN_POINT('Ctrl Pts',(7.76105956129052,-14.8858405817402,-11.1002085369641));
#65488=CARTESIAN_POINT('Ctrl Pts',(7.6384159401128,-14.9141444743334,-10.9707529826629));
#65489=CARTESIAN_POINT('Ctrl Pts',(7.57043047269953,-14.9424536474475,-10.9084183644052));
#65490=CARTESIAN_POINT('Ctrl Pts',(7.5021074297362,-14.9816596935131,-10.8535707098408));
#65491=CARTESIAN_POINT('Ctrl Pts',(7.50105371344569,-14.9822669774523,-10.8527267217707));
#65492=CARTESIAN_POINT('Ctrl Pts',(7.5,-14.9828768864291,-10.8518846384445));
#65493=CARTESIAN_POINT('Origin',(5.75,-11.145178817862,-15.3878195049812));
#65494=CARTESIAN_POINT('Ctrl Pts',(7.5,-10.8518846384445,-14.9828768864291));
#65495=CARTESIAN_POINT('Ctrl Pts',(7.50105371344605,-10.852726721771,-14.9822669774521));
#65496=CARTESIAN_POINT('Ctrl Pts',(7.5021074297361,-10.8535707098409,-14.981659693513));
#65497=CARTESIAN_POINT('Ctrl Pts',(7.59351569467807,-10.9269504763458,-14.9292065753494));
#65498=CARTESIAN_POINT('Ctrl Pts',(7.68214848767641,-11.0120989243862,-14.8976245327993));
#65499=CARTESIAN_POINT('Ctrl Pts',(7.81958013152834,-11.1704454530309,-14.8836434033438));
#65500=CARTESIAN_POINT('Ctrl Pts',(7.87098023972501,-11.2398826207744,-14.8919941158642));
#65501=CARTESIAN_POINT('Ctrl Pts',(7.94048867507028,-11.3545161973503,-14.930821569437));
#65502=CARTESIAN_POINT('Ctrl Pts',(7.96491477585457,-11.4033401554801,-14.9558097197836));
#65503=CARTESIAN_POINT('Ctrl Pts',(7.98678347589508,-11.4662908869419,-15.0039319604953));
#65504=CARTESIAN_POINT('Ctrl Pts',(7.99147733125719,-11.4829744844687,-15.0185083904015));
#65505=CARTESIAN_POINT('Ctrl Pts',(7.99471483544825,-11.4987322084552,-15.034266114388));
#65506=CARTESIAN_POINT('Origin',(7.5,0.,0.));
#65507=CARTESIAN_POINT('Origin',(8.,0.,0.));
#65508=CARTESIAN_POINT('Origin',(8.,-13.3643181644258,-13.3643181644257));
#65509=CARTESIAN_POINT('Origin',(8.,-15.556349186104,12.0208152801713));
#65510=CARTESIAN_POINT('Origin',(8.,15.556349186104,-12.0208152801713));
#65511=CARTESIAN_POINT('',(25.5,14.7292483497821,-11.1937144438494));
#65512=CARTESIAN_POINT('Origin',(25.5,0.,0.));
#65513=CARTESIAN_POINT('Origin',(25.5,0.,0.));
#65514=CARTESIAN_POINT('Origin',(-6.5,21.5,3.5));
#65515=CARTESIAN_POINT('Origin',(-6.25,0.,0.));
#65516=CARTESIAN_POINT('Origin',(-6.25,0.,0.));
#65549=UNCERTAINTY_MEASURE_WITH_UNIT(LENGTH_MEASURE(0.01),#65564,
'DISTANCE_ACCURACY_VALUE',
'Maximum model space distance between geometric entities at asserted c
onnectivities');
#65550=UNCERTAINTY_MEASURE_WITH_UNIT(LENGTH_MEASURE(0.01),#65564,
'DISTANCE_ACCURACY_VALUE',
'Maximum model space distance between geometric entities at asserted c
onnectivities');
#65562=(
GEOMETRIC_REPRESENTATION_CONTEXT(3)
GLOBAL_UNCERTAINTY_ASSIGNED_CONTEXT((#65549))
GLOBAL_UNIT_ASSIGNED_CONTEXT((#65564,#65566,#65567))
REPRESENTATION_CONTEXT('','3D')
);
#65563=(
GEOMETRIC_REPRESENTATION_CONTEXT(3)
GLOBAL_UNCERTAINTY_ASSIGNED_CONTEXT((#65550))
GLOBAL_UNIT_ASSIGNED_CONTEXT((#65564,#65566,#65567))
REPRESENTATION_CONTEXT('','3D')
);
#65564=(
LENGTH_UNIT()
NAMED_UNIT(*)
SI_UNIT(.MILLI.,.METRE.)
);
#65566=(
NAMED_UNIT(*)
PLANE_ANGLE_UNIT()
SI_UNIT($,.RADIAN.)
);
#65567=(
NAMED_UNIT(*)
SI_UNIT($,.STERADIAN.)
SOLID_ANGLE_UNIT()
);
#65579=SHAPE_DEFINITION_REPRESENTATION(#65591,#65624);
#65591=PRODUCT_DEFINITION_SHAPE('',$,#65637);
#65624=SHAPE_REPRESENTATION('',(#22041),#65562);
#65625=PRODUCT_DEFINITION_CONTEXT('part definition',#65663,'design');
#65637=PRODUCT_DEFINITION('2026-10-10-05-45-31-198',
'11_Brass_Driver_Sleeve',#65649,#65625);
#65649=PRODUCT_DEFINITION_FORMATION('',$,#65676);
#65663=APPLICATION_CONTEXT(
'Core Data for Automotive Mechanical Design Process');
#65664=PRODUCT_CONTEXT('part definition',#65663,'mechanical');
#65676=PRODUCT('2026-10-10-05-45-31-198','11_Brass_Driver_Sleeve',$,(#65664));
#65796=COLOUR_RGB('Off White',0.89,0.88,0.83);
#65797=FILL_AREA_STYLE_COLOUR('',#65796);
#65798=FILL_AREA_STYLE('',(#65797));
#65799=SURFACE_STYLE_FILL_AREA(#65798);
#65800=SURFACE_SIDE_STYLE('',(#65799));
#65801=SURFACE_STYLE_USAGE(.BOTH.,#65800);
#65802=PRESENTATION_STYLE_ASSIGNMENT((#65801));
ENDSEC;
END-ISO-10303-21;
